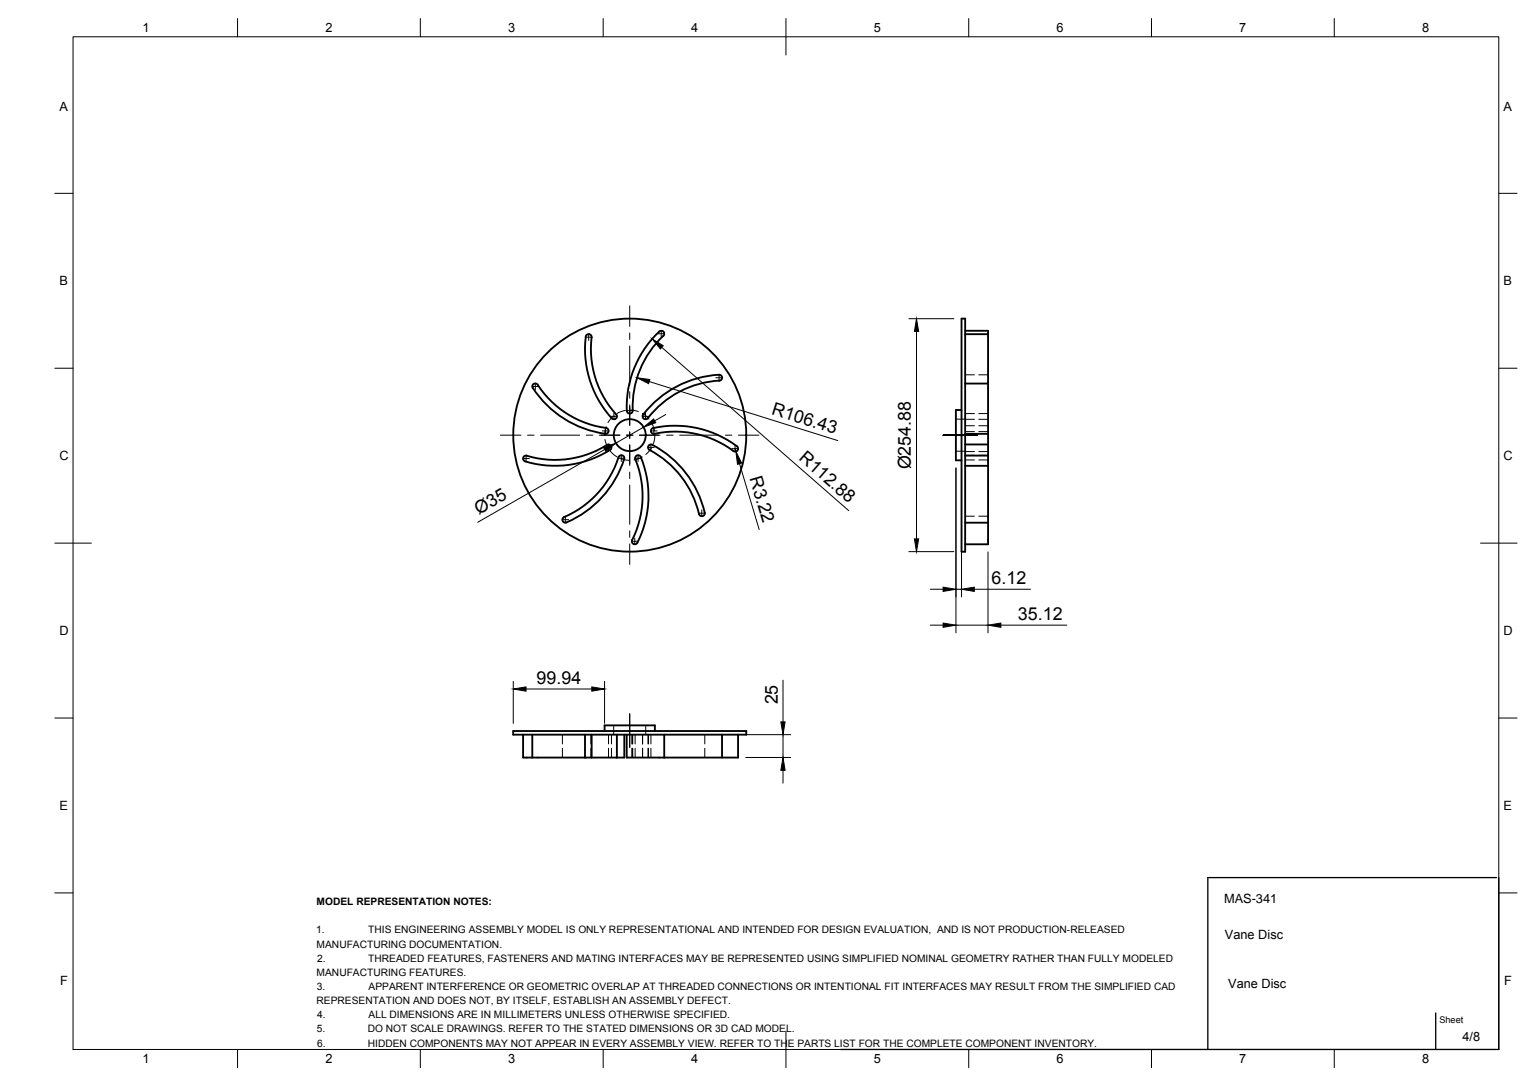
ISO-10303-21;
HEADER;
FILE_DESCRIPTION (('STEP AP214'),
    '1' );
FILE_NAME ('Vane Disc.step',
    '2026-10-08T00:39:10',
    ( '' ),
    ( '' ),
    'SwSTEP 2.0',
    'SolidWorks 2025',
    '' );
FILE_SCHEMA (( 'AUTOMOTIVE_DESIGN' ));
ENDSEC;

DATA;
#15=VECTOR ( 'NONE', #9741, 1000.000000000000000 ) ;
#47=AXIS2_PLACEMENT_3D ( 'NONE', #14477, #18892, #8730 ) ;
#49=ORIENTED_EDGE ( 'NONE', *, *, #19031, .T. ) ;
#59=LINE ( 'NONE', #18583, #13084 ) ;
#66=ORIENTED_EDGE ( 'NONE', *, *, #9551, .T. ) ;
#69=CARTESIAN_POINT ( 'NONE',  ( 57.41881860123199743, 83.27814316901175573, 14.88498244535504966 ) ) ;
#78=DIRECTION ( 'NONE',  ( 0.4999999999999920619, -0.8660254037844431485, -3.488064225688951427E-15 ) ) ;
#89=CARTESIAN_POINT ( 'NONE',  ( 9.176097008933345123, -25.21111933077053990, 14.88498244535538895 ) ) ;
#105=ADVANCED_FACE ( 'NONE', ( #15832 ), #1708, .T. ) ;
#111=FACE_OUTER_BOUND ( 'NONE', #19672, .T. ) ;
#131=DIRECTION ( 'NONE',  ( -0.1736481776669408228, -0.9848077530122062440, 2.152196535136390085E-15 ) ) ;
#138=CARTESIAN_POINT ( 'NONE',  ( -19.79297637435821500, 18.57624240429758800, 39.88498244535558968 ) ) ;
#141=VERTEX_POINT ( 'NONE', #14296 ) ;
#193=ORIENTED_EDGE ( 'NONE', *, *, #1304, .F. ) ;
#227=CIRCLE ( 'NONE', #11655, 3.224098631618461663 ) ;
#235=DIRECTION ( 'NONE',  ( 6.982962677686266711E-15, -0.000000000000000000, 1.000000000000000000 ) ) ;
#236=VECTOR ( 'NONE', #1051, 1000.000000000000000 ) ;
#239=CARTESIAN_POINT ( 'NONE',  ( 23.23469325536214214, -13.41455640552199924, 14.88498244535528947 ) ) ;
#259=PLANE ( 'NONE',  #6247 ) ;
#283=DIRECTION ( 'NONE',  ( 6.982962677686266711E-15, -0.000000000000000000, 1.000000000000000000 ) ) ;
#295=VERTEX_POINT ( 'NONE', #16702 ) ;
#302=CIRCLE ( 'NONE', #17951, 3.224098631618462552 ) ;
#306=LINE ( 'NONE', #12370, #13574 ) ;
#313=FACE_OUTER_BOUND ( 'NONE', #5653, .T. ) ;
#315=VERTEX_POINT ( 'NONE', #3550 ) ;
#316=DIRECTION ( 'NONE',  ( -1.000000000000000000, 0.000000000000000000, 6.976128451377902853E-15 ) ) ;
#334=CARTESIAN_POINT ( 'NONE',  ( 113.3640620605769413, -25.59923667990641150, 14.88498244535466064 ) ) ;
#354=CIRCLE ( 'NONE', #18993, 3.224098631618460331 ) ;
#362=DIRECTION ( 'NONE',  ( 6.982962677686266711E-15, -0.000000000000000000, 1.000000000000000000 ) ) ;
#368=ORIENTED_EDGE ( 'NONE', *, *, #19103, .F. ) ;
#379=DIRECTION ( 'NONE',  ( -6.982962677686266711E-15, 0.000000000000000000, -1.000000000000000000 ) ) ;
#390=CYLINDRICAL_SURFACE ( 'NONE', #8511, 3.224098631618460331 ) ;
#428=AXIS2_PLACEMENT_3D ( 'NONE', #8906, #8812, #13303 ) ;
#429=AXIS2_PLACEMENT_3D ( 'NONE', #16436, #7119, #13337 ) ;
#441=FACE_OUTER_BOUND ( 'NONE', #8088, .T. ) ;
#446=CARTESIAN_POINT ( 'NONE',  ( 19.63382932406841519, 18.38657833536341357, 39.88498244535531967 ) ) ;
#451=AXIS2_PLACEMENT_3D ( 'NONE', #4114, #2798, #845 ) ;
#456=DIRECTION ( 'NONE',  ( -0.7660444431189771253, 0.6427876096865404731, 5.349259755748777816E-15 ) ) ;
#460=AXIS2_PLACEMENT_3D ( 'NONE', #12907, #17728, #3504 ) ;
#465=CIRCLE ( 'NONE', #17772, 3.224098631618455890 ) ;
#466=FACE_OUTER_BOUND ( 'NONE', #14778, .T. ) ;
#478=EDGE_CURVE ( 'NONE', #6273, #3496, #1532, .T. ) ;
#485=CYLINDRICAL_SURFACE ( 'NONE', #1937, 3.224098631618460331 ) ;
#501=CIRCLE ( 'NONE', #1476, 17.50000000000000355 ) ;
#504=AXIS2_PLACEMENT_3D ( 'NONE', #6795, #13106, #738 ) ;
#520=EDGE_CURVE ( 'NONE', #7250, #912, #6769, .T. ) ;
#528=EDGE_LOOP ( 'NONE', ( #18695, #4336, #8989, #6164 ) ) ;
#533=AXIS2_PLACEMENT_3D ( 'NONE', #16138, #2125, #78 ) ;
#538=DIRECTION ( 'NONE',  ( 1.000000000000000000, 0.000000000000000000, -6.994638739193269649E-15 ) ) ;
#562=CARTESIAN_POINT ( 'NONE',  ( -32.30548103355237544, 113.3261241031799926, 14.88498244535567672 ) ) ;
#568=LINE ( 'NONE', #2209, #10145 ) ;
#582=AXIS2_PLACEMENT_3D ( 'NONE', #17065, #9285, #15422 ) ;
#612=LINE ( 'NONE', #19529, #7209 ) ;
#613=DIRECTION ( 'NONE',  ( -6.982962677686266711E-15, 0.000000000000000000, -1.000000000000000000 ) ) ;
#619=ORIENTED_EDGE ( 'NONE', *, *, #10225, .F. ) ;
#640=LINE ( 'NONE', #13102, #7507 ) ;
#641=CARTESIAN_POINT ( 'NONE',  ( -113.3514208120937781, -17.29894464209964866, 14.88498244535624337 ) ) ;
#643=( NAMED_UNIT ( * ) SI_UNIT ( $, .STERADIAN. ) SOLID_ANGLE_UNIT ( ) );
#650=DIRECTION ( 'NONE',  ( -6.982962677686266711E-15, 0.000000000000000000, -1.000000000000000000 ) ) ;
#691=CARTESIAN_POINT ( 'NONE',  ( -34.51244174799990816, 110.9757759606085017, 14.88498244535569093 ) ) ;
#692=DIRECTION ( 'NONE',  ( -0.7660444431189766812, 0.6427876096865408062, 4.304393070272782536E-15 ) ) ;
#724=CIRCLE ( 'NONE', #19044, 3.224098631618458999 ) ;
#732=AXIS2_PLACEMENT_3D ( 'NONE', #11861, #13300, #19653 ) ;
#734=DIRECTION ( 'NONE',  ( -6.982962677686265922E-15, -1.972152263052529514E-31, -1.000000000000000000 ) ) ;
#735=CARTESIAN_POINT ( 'NONE',  ( 23.23469325536214214, -13.41455640552199924, 14.88498244535528947 ) ) ;
#738=DIRECTION ( 'NONE',  ( 0.5000000000000038858, 0.8660254037844363761, -3.520662956770155909E-15 ) ) ;
#745=EDGE_CURVE ( 'NONE', #1745, #14667, #18421, .T. ) ;
#747=ORIENTED_EDGE ( 'NONE', *, *, #8839, .T. ) ;
#749=CARTESIAN_POINT ( 'NONE',  ( 92.34802049131684498, -66.64338626758360817, 14.88498244535480630 ) ) ;
#754=DIRECTION ( 'NONE',  ( 6.982962677686266711E-15, -0.000000000000000000, 1.000000000000000000 ) ) ;
#759=CARTESIAN_POINT ( 'NONE',  ( -26.42151830275515323, 4.658826548058537576, 14.88498244535563586 ) ) ;
#790=CARTESIAN_POINT ( 'NONE',  ( -63.98537287693023501, 94.20918150411493741, 39.88498244535590231 ) ) ;
#792=ORIENTED_EDGE ( 'NONE', *, *, #6721, .T. ) ;
#797=CARTESIAN_POINT ( 'NONE',  ( -9.176097008933940202, -25.21111933077039069, 39.88498244535551862 ) ) ;
#807=VERTEX_POINT ( 'NONE', #18628 ) ;
#818=VERTEX_POINT ( 'NONE', #9309 ) ;
#831=FACE_OUTER_BOUND ( 'NONE', #15190, .T. ) ;
#845=DIRECTION ( 'NONE',  ( 1.000000000000000000, 0.000000000000000000, -6.994638739193269649E-15 ) ) ;
#850=CARTESIAN_POINT ( 'NONE',  ( -63.98537287693023501, 94.20918150411493741, 39.88498244535590231 ) ) ;
#851=ADVANCED_FACE ( 'NONE', ( #5221 ), #6350, .T. ) ;
#863=ORIENTED_EDGE ( 'NONE', *, *, #8888, .F. ) ;
#891=CIRCLE ( 'NONE', #13620, 3.224098631618461663 ) ;
#895=AXIS2_PLACEMENT_3D ( 'NONE', #13323, #2501, #8636 ) ;
#896=EDGE_CURVE ( 'NONE', #12923, #1501, #465, .T. ) ;
#904=EDGE_CURVE ( 'NONE', #2440, #7038, #2047, .T. ) ;
#908=DIRECTION ( 'NONE',  ( 6.982962677686266711E-15, -0.000000000000000000, 1.000000000000000000 ) ) ;
#912=VERTEX_POINT ( 'NONE', #10300 ) ;
#931=CARTESIAN_POINT ( 'NONE',  ( -20.01059462374426445, -13.41455640552162443, 14.88498244535559323 ) ) ;
#936=DIRECTION ( 'NONE',  ( -0.7660444431189770143, 0.6427876096865405842, 5.348151281215662765E-15 ) ) ;
#965=ORIENTED_EDGE ( 'NONE', *, *, #16251, .F. ) ;
#979=AXIS2_PLACEMENT_3D ( 'NONE', #2375, #18027, #5444 ) ;
#981=CARTESIAN_POINT ( 'NONE',  ( 112.4320812185962524, -22.51277856475483574, 14.88498244535466775 ) ) ;
#994=LINE ( 'NONE', #7047, #13321 ) ;
#996=FACE_OUTER_BOUND ( 'NONE', #16761, .T. ) ;
#1003=CARTESIAN_POINT ( 'NONE',  ( -49.59485801383857506, -102.5175491340983882, 14.88498244535579929 ) ) ;
#1008=DIRECTION ( 'NONE',  ( -6.982962677686268288E-15, 3.944304526105059903E-31, -1.000000000000000000 ) ) ;
#1009=ORIENTED_EDGE ( 'NONE', *, *, #7477, .F. ) ;
#1017=VECTOR ( 'NONE', #3317, 1000.000000000000000 ) ;
#1024=CARTESIAN_POINT ( 'NONE',  ( 25.98398601615827985, 7.853099154550822192, 14.88498244535527171 ) ) ;
#1045=ORIENTED_EDGE ( 'NONE', *, *, #5358, .T. ) ;
#1051=DIRECTION ( 'NONE',  ( 6.982962677686266711E-15, -0.000000000000000000, 1.000000000000000000 ) ) ;
#1056=CIRCLE ( 'NONE', #8250, 3.224098631618458555 ) ;
#1060=CIRCLE ( 'NONE', #5338, 27.50000000000000355 ) ;
#1065=AXIS2_PLACEMENT_3D ( 'NONE', #69, #12331, #10906 ) ;
#1066=DIRECTION ( 'NONE',  ( -1.000000000000000000, 0.000000000000000000, 0.000000000000000000 ) ) ;
#1067=CARTESIAN_POINT ( 'NONE',  ( -49.59485801383857506, -102.5175491340983882, 14.88498244535579929 ) ) ;
#1079=CIRCLE ( 'NONE', #19402, 3.224098631618458999 ) ;
#1080=VERTEX_POINT ( 'NONE', #12131 ) ;
#1084=MANIFOLD_SOLID_BREP ( 'Boss-Extrude13', #11640 ) ;
#1110=ORIENTED_EDGE ( 'NONE', *, *, #2464, .F. ) ;
#1134=CARTESIAN_POINT ( 'NONE',  ( -2.647132857508548209, -114.6332882433608376, 14.88498244535546888 ) ) ;
#1136=ORIENTED_EDGE ( 'NONE', *, *, #18917, .F. ) ;
#1170=DIRECTION ( 'NONE',  ( 1.000000000000000000, 0.000000000000000000, -6.977185866873308817E-15 ) ) ;
#1189=AXIS2_PLACEMENT_3D ( 'NONE', #2625, #2520, #15088 ) ;
#1198=CIRCLE ( 'NONE', #19820, 3.224098631618463440 ) ;
#1200=DIRECTION ( 'NONE',  ( 1.000000000000000000, 0.000000000000000000, -6.994638739193269649E-15 ) ) ;
#1209=CARTESIAN_POINT ( 'NONE',  ( -1.396592535537253342E-14, 0.000000000000000000, 39.88498244535545467 ) ) ;
#1225=DIRECTION ( 'NONE',  ( 0.9396926207859057634, -0.3420201433256758183, -6.456589605409169860E-15 ) ) ;
#1235=ORIENTED_EDGE ( 'NONE', *, *, #20238, .T. ) ;
#1236=CYLINDRICAL_SURFACE ( 'NONE', #15630, 112.8770930172170210 ) ;
#1244=AXIS2_PLACEMENT_3D ( 'NONE', #14765, #2203, #19186 ) ;
#1254=DIRECTION ( 'NONE',  ( 6.982962677686266711E-15, 0.000000000000000000, 1.000000000000000000 ) ) ;
#1261=CIRCLE ( 'NONE', #14662, 106.4288957539801004 ) ;
#1264=AXIS2_PLACEMENT_3D ( 'NONE', #6211, #1494, #1695 ) ;
#1290=CARTESIAN_POINT ( 'NONE',  ( 27.50000000000001776, 3.367778697655222096E-15, 49.99999999999998579 ) ) ;
#1301=DIRECTION ( 'NONE',  ( 6.982962677686266711E-15, -0.000000000000000000, 1.000000000000000000 ) ) ;
#1304=EDGE_CURVE ( 'NONE', #6273, #295, #16535, .T. ) ;
#1308=ORIENTED_EDGE ( 'NONE', *, *, #4869, .T. ) ;
#1311=LINE ( 'NONE', #8969, #8332 ) ;
#1316=CARTESIAN_POINT ( 'NONE',  ( -27.49999999999998934, 0.000000000000000000, 49.99999999999998579 ) ) ;
#1331=ORIENTED_EDGE ( 'NONE', *, *, #4320, .F. ) ;
#1340=CYLINDRICAL_SURFACE ( 'NONE', #18052, 3.224098631618460331 ) ;
#1361=CYLINDRICAL_SURFACE ( 'NONE', #13666, 3.224098631618460331 ) ;
#1371=EDGE_CURVE ( 'NONE', #7864, #8547, #19790, .T. ) ;
#1384=CARTESIAN_POINT ( 'NONE',  ( 113.5802308907675666, 8.308367629983374414, 14.88498244535465709 ) ) ;
#1401=VERTEX_POINT ( 'NONE', #10676 ) ;
#1411=ORIENTED_EDGE ( 'NONE', *, *, #10835, .F. ) ;
#1427=EDGE_LOOP ( 'NONE', ( #19804, #8340, #5647, #20218 ) ) ;
#1433=ORIENTED_EDGE ( 'NONE', *, *, #6415, .F. ) ;
#1461=CARTESIAN_POINT ( 'NONE',  ( -14.69786621328394283, 22.52834316112731017, 39.88498244535555415 ) ) ;
#1476=AXIS2_PLACEMENT_3D ( 'NONE', #15111, #17998, #7440 ) ;
#1494=DIRECTION ( 'NONE',  ( 6.982962677686266711E-15, -0.000000000000000000, 1.000000000000000000 ) ) ;
#1495=LINE ( 'NONE', #17151, #9162 ) ;
#1501=VERTEX_POINT ( 'NONE', #15497 ) ;
#1506=ORIENTED_EDGE ( 'NONE', *, *, #8714, .T. ) ;
#1515=AXIS2_PLACEMENT_3D ( 'NONE', #7804, #13076, #3208 ) ;
#1532=CIRCLE ( 'NONE', #13602, 127.4413876050234649 ) ;
#1543=EDGE_CURVE ( 'NONE', #6114, #17930, #5067, .T. ) ;
#1553=CARTESIAN_POINT ( 'NONE',  ( -81.99056186900673993, -84.64042930812179577, 14.88498244535602488 ) ) ;
#1600=ORIENTED_EDGE ( 'NONE', *, *, #3125, .F. ) ;
#1630=CARTESIAN_POINT ( 'NONE',  ( -75.71267875615025389, -86.11264925328200093, 14.88498244535597870 ) ) ;
#1633=DIRECTION ( 'NONE',  ( 6.982962677686266711E-15, -0.000000000000000000, 1.000000000000000000 ) ) ;
#1647=LINE ( 'NONE', #6357, #17013 ) ;
#1648=DIRECTION ( 'NONE',  ( -6.982962677686266711E-15, 0.000000000000000000, -1.000000000000000000 ) ) ;
#1654=DIRECTION ( 'NONE',  ( 6.982962677686266711E-15, -0.000000000000000000, 1.000000000000000000 ) ) ;
#1671=CARTESIAN_POINT ( 'NONE',  ( -2.300765332208190905, -116.0870680293436408, 39.88498244535547599 ) ) ;
#1676=CARTESIAN_POINT ( 'NONE',  ( 27.50000000000001776, 3.367778697655222096E-15, 43.88498244535526993 ) ) ;
#1694=DIRECTION ( 'NONE',  ( 6.982962677686266711E-15, -0.000000000000000000, 1.000000000000000000 ) ) ;
#1695=DIRECTION ( 'NONE',  ( 1.000000000000000000, 0.000000000000000000, -6.977185866873308817E-15 ) ) ;
#1696=CARTESIAN_POINT ( 'NONE',  ( -19.79297637435836421, 18.57624240429761642, 14.88498244535559145 ) ) ;
#1698=ORIENTED_EDGE ( 'NONE', *, *, #16107, .F. ) ;
#1708=CYLINDRICAL_SURFACE ( 'NONE', #3475, 3.224098631618460331 ) ;
#1727=AXIS2_PLACEMENT_3D ( 'NONE', #16670, #1633, #18506 ) ;
#1733=DIRECTION ( 'NONE',  ( 1.000000000000000000, 0.000000000000000000, -6.977185866873309606E-15 ) ) ;
#1743=DIRECTION ( 'NONE',  ( 6.982962677686266711E-15, -0.000000000000000000, 1.000000000000000000 ) ) ;
#1745=VERTEX_POINT ( 'NONE', #562 ) ;
#1748=CARTESIAN_POINT ( 'NONE',  ( -6.191009641800430785, -26.42934155884822900, 14.88498244535549375 ) ) ;
#1760=ORIENTED_EDGE ( 'NONE', *, *, #17363, .F. ) ;
#1763=MECHANICAL_DESIGN_GEOMETRIC_PRESENTATION_REPRESENTATION('',(#18100),#5359);
#1777=CIRCLE ( 'NONE', #8629, 3.224098631618458999 ) ;
#1797=DIRECTION ( 'NONE',  ( 0.5000000000000038858, 0.8660254037844362651, -3.503961184244744203E-15 ) ) ;
#1799=FACE_BOUND ( 'NONE', #7536, .T. ) ;
#1801=DIRECTION ( 'NONE',  ( 6.982962677686266711E-15, -0.000000000000000000, 1.000000000000000000 ) ) ;
#1807=VERTEX_POINT ( 'NONE', #16606 ) ;
#1814=AXIS2_PLACEMENT_3D ( 'NONE', #14717, #19236, #2052 ) ;
#1824=AXIS2_PLACEMENT_3D ( 'NONE', #9990, #3945, #13342 ) ;
#1830=ORIENTED_EDGE ( 'NONE', *, *, #7477, .T. ) ;
#1839=ORIENTED_EDGE ( 'NONE', *, *, #16386, .F. ) ;
#1862=VERTEX_POINT ( 'NONE', #4019 ) ;
#1874=VECTOR ( 'NONE', #18951, 1000.000000000000000 ) ;
#1877=FACE_OUTER_BOUND ( 'NONE', #6342, .T. ) ;
#1891=EDGE_CURVE ( 'NONE', #1401, #4820, #9815, .T. ) ;
#1898=CARTESIAN_POINT ( 'NONE',  ( -81.99056186900673993, -84.64042930812179577, 14.88498244535602488 ) ) ;
#1900=DIRECTION ( 'NONE',  ( -0.1736481776669404620, -0.9848077530122062440, 1.229460064647279239E-15 ) ) ;
#1902=CIRCLE ( 'NONE', #9740, 3.224098631618460331 ) ;
#1911=EDGE_LOOP ( 'NONE', ( #19538, #3190 ) ) ;
#1918=CIRCLE ( 'NONE', #18576, 3.224098631618463440 ) ;
#1937=AXIS2_PLACEMENT_3D ( 'NONE', #10093, #14596, #6729 ) ;
#1944=LINE ( 'NONE', #8173, #2255 ) ;
#1946=CARTESIAN_POINT ( 'NONE',  ( 1.396592535537252080E-14, 0.000000000000000000, 49.99999999999998579 ) ) ;
#1956=DIRECTION ( 'NONE',  ( -6.982962677686266711E-15, 0.000000000000000000, -1.000000000000000000 ) ) ;
#1980=AXIS2_PLACEMENT_3D ( 'NONE', #4506, #9206, #7367 ) ;
#1986=PLANE ( 'NONE',  #4620 ) ;
#1994=VERTEX_POINT ( 'NONE', #11245 ) ;
#2003=CIRCLE ( 'NONE', #17696, 3.224098631618460331 ) ;
#2009=ORIENTED_EDGE ( 'NONE', *, *, #9610, .T. ) ;
#2014=VERTEX_POINT ( 'NONE', #641 ) ;
#2023=DIRECTION ( 'NONE',  ( 1.000000000000000000, 0.000000000000000000, -6.977185866873308817E-15 ) ) ;
#2024=ORIENTED_EDGE ( 'NONE', *, *, #9144, .F. ) ;
#2027=CARTESIAN_POINT ( 'NONE',  ( 103.2967819461769921, 53.25886146954521649, 39.88498244535472992 ) ) ;
#2034=DIRECTION ( 'NONE',  ( 6.982962677686266711E-15, -0.000000000000000000, 1.000000000000000000 ) ) ;
#2036=DIRECTION ( 'NONE',  ( -6.982962677686266711E-15, 0.000000000000000000, -1.000000000000000000 ) ) ;
#2047=LINE ( 'NONE', #8277, #14496 ) ;
#2050=EDGE_CURVE ( 'NONE', #16647, #4108, #4200, .T. ) ;
#2052=DIRECTION ( 'NONE',  ( -1.000000000000000000, 0.000000000000000000, 6.969309079188926949E-15 ) ) ;
#2053=CARTESIAN_POINT ( 'NONE',  ( -12.16118437606778535, -23.99289710269258080, 14.88498244535553461 ) ) ;
#2069=ORIENTED_EDGE ( 'NONE', *, *, #9873, .T. ) ;
#2086=AXIS2_PLACEMENT_3D ( 'NONE', #790, #13357, #2531 ) ;
#2089=DIRECTION ( 'NONE',  ( -6.982962677686266711E-15, 0.000000000000000000, -1.000000000000000000 ) ) ;
#2115=CIRCLE ( 'NONE', #14846, 112.8770930172170353 ) ;
#2125=DIRECTION ( 'NONE',  ( 6.982962677686266711E-15, 0.000000000000000000, 1.000000000000000000 ) ) ;
#2138=EDGE_LOOP ( 'NONE', ( #12512, #19684, #12449, #17623, #12034 ) ) ;
#2156=CYLINDRICAL_SURFACE ( 'NONE', #1515, 112.8770930172170068 ) ;
#2159=DIRECTION ( 'NONE',  ( 1.000000000000000000, 0.000000000000000000, -6.977185866873308817E-15 ) ) ;
#2163=DIRECTION ( 'NONE',  ( 1.000000000000000000, 0.000000000000000000, -6.994638739193269649E-15 ) ) ;
#2170=VERTEX_POINT ( 'NONE', #15944 ) ;
#2171=AXIS2_PLACEMENT_3D ( 'NONE', #7203, #10261, #7102 ) ;
#2184=VERTEX_POINT ( 'NONE', #17783 ) ;
#2195=CIRCLE ( 'NONE', #1189, 3.224098631618460331 ) ;
#2199=DIRECTION ( 'NONE',  ( 6.982962677686266711E-15, -0.000000000000000000, 1.000000000000000000 ) ) ;
#2203=DIRECTION ( 'NONE',  ( 6.982962677686266711E-15, -0.000000000000000000, 1.000000000000000000 ) ) ;
#2209=CARTESIAN_POINT ( 'NONE',  ( 6.106329265062790945, -26.19668413589285194, 14.88498244535541026 ) ) ;
#2212=VECTOR ( 'NONE', #12651, 1000.000000000000000 ) ;
#2213=ORIENTED_EDGE ( 'NONE', *, *, #9199, .F. ) ;
#2214=AXIS2_PLACEMENT_3D ( 'NONE', #13685, #4382, #20133 ) ;
#2217=ORIENTED_EDGE ( 'NONE', *, *, #7018, .F. ) ;
#2220=EDGE_LOOP ( 'NONE', ( #965, #6524, #11975, #17424 ) ) ;
#2227=ORIENTED_EDGE ( 'NONE', *, *, #10835, .T. ) ;
#2251=EDGE_CURVE ( 'NONE', #12128, #7331, #354, .T. ) ;
#2255=VECTOR ( 'NONE', #17295, 1000.000000000000000 ) ;
#2256=AXIS2_PLACEMENT_3D ( 'NONE', #2903, #17019, #2801 ) ;
#2259=DIRECTION ( 'NONE',  ( 1.000000000000000000, 0.000000000000000000, -6.976128451377902853E-15 ) ) ;
#2261=ORIENTED_EDGE ( 'NONE', *, *, #19165, .T. ) ;
#2262=CARTESIAN_POINT ( 'NONE',  ( 43.41157826374501383, -91.36522714846361737, 14.88498244535515092 ) ) ;
#2286=DIRECTION ( 'NONE',  ( -0.1736481776669280275, 0.9848077530122084644, 1.076098267568195831E-15 ) ) ;
#2287=FACE_OUTER_BOUND ( 'NONE', #13566, .T. ) ;
#2292=EDGE_LOOP ( 'NONE', ( #11795, #6552, #5825, #9650, #2390 ) ) ;
#2308=DIRECTION ( 'NONE',  ( -6.982962677686266711E-15, 0.000000000000000000, -1.000000000000000000 ) ) ;
#2334=LINE ( 'NONE', #5907, #5129 ) ;
#2341=VERTEX_POINT ( 'NONE', #5591 ) ;
#2356=PLANE ( 'NONE',  #15439 ) ;
#2368=ORIENTED_EDGE ( 'NONE', *, *, #3905, .T. ) ;
#2372=AXIS2_PLACEMENT_3D ( 'NONE', #11461, #15974, #14437 ) ;
#2375=CARTESIAN_POINT ( 'NONE',  ( 26.42151830275502178, 4.658826548058130790, 39.88498244535526993 ) ) ;
#2378=( NAMED_UNIT ( * ) PLANE_ANGLE_UNIT ( ) SI_UNIT ( $, .RADIAN. ) );
#2385=VECTOR ( 'NONE', #9210, 1000.000000000000000 ) ;
#2390=ORIENTED_EDGE ( 'NONE', *, *, #8482, .T. ) ;
#2409=VERTEX_POINT ( 'NONE', #12117 ) ;
#2426=VERTEX_POINT ( 'NONE', #17253 ) ;
#2432=CARTESIAN_POINT ( 'NONE',  ( -78.85162031257850401, -85.37653928070189124, 14.88498244535600357 ) ) ;
#2440=VERTEX_POINT ( 'NONE', #1290 ) ;
#2452=FACE_OUTER_BOUND ( 'NONE', #7683, .T. ) ;
#2464=EDGE_CURVE ( 'NONE', #1862, #16627, #2003, .T. ) ;
#2466=CARTESIAN_POINT ( 'NONE',  ( -23.23469325536272478, -13.41455640552162443, 14.88498244535561454 ) ) ;
#2476=DIRECTION ( 'NONE',  ( 0.5000000000000044409, 0.8660254037844360431, -3.228294802704586902E-15 ) ) ;
#2477=CARTESIAN_POINT ( 'NONE',  ( -19.79297637435836421, 18.57624240429761642, 14.88498244535559145 ) ) ;
#2482=DIRECTION ( 'NONE',  ( -6.982962677686266711E-15, 0.000000000000000000, -1.000000000000000000 ) ) ;
#2493=LINE ( 'NONE', #14864, #17654 ) ;
#2499=EDGE_CURVE ( 'NONE', #6452, #10937, #9506, .T. ) ;
#2501=DIRECTION ( 'NONE',  ( 6.982962677686266711E-15, 0.000000000000000000, 1.000000000000000000 ) ) ;
#2504=VECTOR ( 'NONE', #6931, 1000.000000000000000 ) ;
#2506=AXIS2_PLACEMENT_3D ( 'NONE', #2466, #14836, #18114 ) ;
#2513=DIRECTION ( 'NONE',  ( 6.982962677686266711E-15, -0.000000000000000000, 1.000000000000000000 ) ) ;
#2520=DIRECTION ( 'NONE',  ( -6.982962677686266711E-15, 0.000000000000000000, -1.000000000000000000 ) ) ;
#2531=DIRECTION ( 'NONE',  ( -0.7660444431189770143, 0.6427876096865404731, 5.348151281215661977E-15 ) ) ;
#2532=EDGE_LOOP ( 'NONE', ( #16841, #13833, #9327, #7473 ) ) ;
#2538=CIRCLE ( 'NONE', #8424, 3.224098631618455890 ) ;
#2555=VERTEX_POINT ( 'NONE', #14581 ) ;
#2556=CIRCLE ( 'NONE', #18580, 106.4288957539801004 ) ;
#2562=CARTESIAN_POINT ( 'NONE',  ( 3.304959094393253416, 31.03941509555038181, 14.88498244535543158 ) ) ;
#2580=DIRECTION ( 'NONE',  ( -1.000000000000000000, 0.000000000000000000, 6.994638739193269649E-15 ) ) ;
#2589=EDGE_CURVE ( 'NONE', #19558, #4614, #11097, .T. ) ;
#2593=CARTESIAN_POINT ( 'NONE',  ( -109.5721339228237667, 31.03941509555038181, 14.88498244535621851 ) ) ;
#2597=DIRECTION ( 'NONE',  ( 6.982962677686266711E-15, 0.000000000000000000, 1.000000000000000000 ) ) ;
#2614=EDGE_LOOP ( 'NONE', ( #3626, #14039, #11730, #7222 ) ) ;
#2623=LINE ( 'NONE', #6930, #20205 ) ;
#2625=CARTESIAN_POINT ( 'NONE',  ( -17.24542129382105315, 20.55229278271246329, 39.88498244535557546 ) ) ;
#2628=CIRCLE ( 'NONE', #6555, 112.8770930172170495 ) ;
#2632=DIRECTION ( 'NONE',  ( 0.000000000000000000, 0.000000000000000000, 1.000000000000000000 ) ) ;
#2634=LINE ( 'NONE', #8859, #18820 ) ;
#2636=EDGE_LOOP ( 'NONE', ( #12071, #6685, #2683, #19660 ) ) ;
#2652=DIRECTION ( 'NONE',  ( 6.982962677686266711E-15, -0.000000000000000000, 1.000000000000000000 ) ) ;
#2665=EDGE_CURVE ( 'NONE', #807, #11267, #3835, .T. ) ;
#2670=ORIENTED_EDGE ( 'NONE', *, *, #11507, .T. ) ;
#2676=CARTESIAN_POINT ( 'NONE',  ( -14.02132266220259460, 20.55229278271246329, 39.88498244535555415 ) ) ;
#2679=DIRECTION ( 'NONE',  ( -0.7660444431189766812, 0.6427876096865408062, 5.380491337840978959E-15 ) ) ;
#2682=LINE ( 'NONE', #19756, #12827 ) ;
#2683=ORIENTED_EDGE ( 'NONE', *, *, #11372, .F. ) ;
#2700=VECTOR ( 'NONE', #10838, 1000.000000000000000 ) ;
#2707=ORIENTED_EDGE ( 'NONE', *, *, #11874, .T. ) ;
#2722=DIRECTION ( 'NONE',  ( -6.982962677686266711E-15, 0.000000000000000000, -1.000000000000000000 ) ) ;
#2727=EDGE_CURVE ( 'NONE', #10937, #7509, #17898, .T. ) ;
#2738=FACE_OUTER_BOUND ( 'NONE', #2292, .T. ) ;
#2782=EDGE_CURVE ( 'NONE', #818, #10937, #15071, .T. ) ;
#2786=VERTEX_POINT ( 'NONE', #5774 ) ;
#2798=DIRECTION ( 'NONE',  ( 6.982962677686266711E-15, -0.000000000000000000, 1.000000000000000000 ) ) ;
#2801=DIRECTION ( 'NONE',  ( -0.7660444431189858960, -0.6427876096865299260, 5.348151281215661977E-15 ) ) ;
#2817=ORIENTED_EDGE ( 'NONE', *, *, #18917, .T. ) ;
#2823=DIRECTION ( 'NONE',  ( 0.9396926207859058744, -0.3420201433256757628, -6.568644312862837946E-15 ) ) ;
#2832=DIRECTION ( 'NONE',  ( 0.9396926207859057634, -0.3420201433256758183, -6.456589605409169860E-15 ) ) ;
#2834=ADVANCED_FACE ( 'NONE', ( #15591 ), #4751, .T. ) ;
#2860=FACE_BOUND ( 'NONE', #7834, .T. ) ;
#2880=DIRECTION ( 'NONE',  ( 6.982962677686266711E-15, -0.000000000000000000, 1.000000000000000000 ) ) ;
#2903=CARTESIAN_POINT ( 'NONE',  ( -103.8888757476053541, -46.65403860089418941, 14.88498244535617765 ) ) ;
#2917=AXIS2_PLACEMENT_3D ( 'NONE', #13299, #10333, #11860 ) ;
#2918=VERTEX_POINT ( 'NONE', #17128 ) ;
#2929=CARTESIAN_POINT ( 'NONE',  ( 9.176097008933345123, -25.21111933077053990, 14.88498244535538895 ) ) ;
#2930=FACE_OUTER_BOUND ( 'NONE', #5894, .T. ) ;
#2935=DIRECTION ( 'NONE',  ( 6.982962677686266711E-15, -0.000000000000000000, 1.000000000000000000 ) ) ;
#2940=DIRECTION ( 'NONE',  ( 0.9396926207859104263, 0.3420201433256629953, -6.562243095054850434E-15 ) ) ;
#2948=FILL_AREA_STYLE_COLOUR ( '', #12204 ) ;
#2982=CARTESIAN_POINT ( 'NONE',  ( -113.3514208120937781, -17.29894464209964866, 14.88498244535624337 ) ) ;
#2987=ADVANCED_FACE ( 'NONE', ( #11483, #9746 ), #1986, .T. ) ;
#3002=EDGE_CURVE ( 'NONE', #3496, #6917, #17341, .T. ) ;
#3036=CARTESIAN_POINT ( 'NONE',  ( 9.176097008933519206, -25.21111933077053990, 39.88498244535539072 ) ) ;
#3046=ADVANCED_FACE ( 'NONE', ( #1877 ), #3212, .T. ) ;
#3054=DIRECTION ( 'NONE',  ( -0.1736481776669405452, -0.9848077530122062440, 1.214091813839188261E-15 ) ) ;
#3056=CYLINDRICAL_SURFACE ( 'NONE', #11893, 3.224098631618457667 ) ;
#3068=CARTESIAN_POINT ( 'NONE',  ( 113.3640620605769413, -25.59923667990641150, 14.88498244535466064 ) ) ;
#3077=CIRCLE ( 'NONE', #8939, 3.224098631618458555 ) ;
#3088=VERTEX_POINT ( 'NONE', #4961 ) ;
#3099=ORIENTED_EDGE ( 'NONE', *, *, #14653, .F. ) ;
#3116=VERTEX_POINT ( 'NONE', #5257 ) ;
#3119=EDGE_CURVE ( 'NONE', #9562, #315, #302, .T. ) ;
#3125=EDGE_CURVE ( 'NONE', #11508, #15057, #9778, .T. ) ;
#3134=DIRECTION ( 'NONE',  ( 1.000000000000000000, 0.000000000000000000, -6.969309079188926949E-15 ) ) ;
#3153=CYLINDRICAL_SURFACE ( 'NONE', #7761, 112.8770930172170210 ) ;
#3165=CIRCLE ( 'NONE', #14589, 3.224098631618458555 ) ;
#3190=ORIENTED_EDGE ( 'NONE', *, *, #7762, .T. ) ;
#3191=AXIS2_PLACEMENT_3D ( 'NONE', #9188, #5107, #10924 ) ;
#3194=AXIS2_PLACEMENT_3D ( 'NONE', #15486, #17025, #18351 ) ;
#3196=EDGE_LOOP ( 'NONE', ( #17005, #17105, #18751, #747, #18294, #2069 ) ) ;
#3202=VERTEX_POINT ( 'NONE', #2477 ) ;
#3208=DIRECTION ( 'NONE',  ( 1.000000000000000000, 0.000000000000000000, -6.977185866873309606E-15 ) ) ;
#3212=CYLINDRICAL_SURFACE ( 'NONE', #5592, 3.224098631618457667 ) ;
#3224=DIRECTION ( 'NONE',  ( 1.000000000000000000, 0.000000000000000000, -6.976128451377903642E-15 ) ) ;
#3227=DIRECTION ( 'NONE',  ( 1.000000000000000000, 0.000000000000000000, -6.994638739193269649E-15 ) ) ;
#3230=DIRECTION ( 'NONE',  ( 6.982962677686266711E-15, 0.000000000000000000, 1.000000000000000000 ) ) ;
#3237=ADVANCED_FACE ( 'NONE', ( #831 ), #6984, .T. ) ;
#3272=EDGE_CURVE ( 'NONE', #8591, #18684, #15440, .T. ) ;
#3278=DIRECTION ( 'NONE',  ( 1.000000000000000000, 0.000000000000000000, -6.994638739193269649E-15 ) ) ;
#3284=DIRECTION ( 'NONE',  ( 6.982962677686266711E-15, -0.000000000000000000, 1.000000000000000000 ) ) ;
#3286=DIRECTION ( 'NONE',  ( -6.982962677686266711E-15, 0.000000000000000000, -1.000000000000000000 ) ) ;
#3291=CYLINDRICAL_SURFACE ( 'NONE', #13183, 106.4288957539801004 ) ;
#3312=DIRECTION ( 'NONE',  ( 1.000000000000000000, 0.000000000000000000, -6.976128451377902853E-15 ) ) ;
#3317=DIRECTION ( 'NONE',  ( 6.982962677686266711E-15, -0.000000000000000000, 1.000000000000000000 ) ) ;
#3319=ORIENTED_EDGE ( 'NONE', *, *, #2589, .F. ) ;
#3322=AXIS2_PLACEMENT_3D ( 'NONE', #13528, #18053, #16618 ) ;
#3337=PLANE ( 'NONE',  #9029 ) ;
#3339=ORIENTED_EDGE ( 'NONE', *, *, #9551, .F. ) ;
#3369=AXIS2_PLACEMENT_3D ( 'NONE', #8959, #1301, #5805 ) ;
#3375=CARTESIAN_POINT ( 'NONE',  ( -5.524863963826822655, -116.0870680293436408, 14.88498244535549020 ) ) ;
#3381=EDGE_CURVE ( 'NONE', #1807, #11267, #9004, .T. ) ;
#3383=AXIS2_PLACEMENT_3D ( 'NONE', #749, #2199, #19286 ) ;
#3423=ADVANCED_FACE ( 'NONE', ( #111 ), #3291, .F. ) ;
#3425=EDGE_LOOP ( 'NONE', ( #16382, #14638, #12899, #18330 ) ) ;
#3445=ORIENTED_EDGE ( 'NONE', *, *, #16774, .F. ) ;
#3459=CIRCLE ( 'NONE', #13569, 112.8770930172170210 ) ;
#3474=CARTESIAN_POINT ( 'NONE',  ( 25.98398601615845038, 7.853099154550832850, 39.88498244535526993 ) ) ;
#3475=AXIS2_PLACEMENT_3D ( 'NONE', #14393, #4992, #17061 ) ;
#3477=ORIENTED_EDGE ( 'NONE', *, *, #14791, .T. ) ;
#3480=AXIS2_PLACEMENT_3D ( 'NONE', #4157, #16644, #16452 ) ;
#3482=ADVANCED_FACE ( 'NONE', ( #313 ), #3592, .T. ) ;
#3488=CARTESIAN_POINT ( 'NONE',  ( -1.396592535537253342E-14, 0.000000000000000000, 39.88498244535545467 ) ) ;
#3496=VERTEX_POINT ( 'NONE', #11051 ) ;
#3504=DIRECTION ( 'NONE',  ( 0.4999999999999925060, -0.8660254037844429265, -4.304393070272789636E-15 ) ) ;
#3506=LINE ( 'NONE', #12910, #15 ) ;
#3547=ORIENTED_EDGE ( 'NONE', *, *, #1891, .T. ) ;
#3548=CIRCLE ( 'NONE', #14966, 3.224098631618461219 ) ;
#3550=CARTESIAN_POINT ( 'NONE',  ( 24.95276293194433492, -10.68636129284900704, 14.88498244535527881 ) ) ;
#3564=DIRECTION ( 'NONE',  ( 1.000000000000000000, 0.000000000000000000, -6.994638739193269649E-15 ) ) ;
#3592=CYLINDRICAL_SURFACE ( 'NONE', #9800, 127.4413876050234649 ) ;
#3594=ORIENTED_EDGE ( 'NONE', *, *, #745, .F. ) ;
#3598=CIRCLE ( 'NONE', #2256, 112.8770930172170637 ) ;
#3612=DIRECTION ( 'NONE',  ( -6.982962677686266711E-15, 0.000000000000000000, -1.000000000000000000 ) ) ;
#3618=CARTESIAN_POINT ( 'NONE',  ( -5.524863963826822655, -116.0870680293436408, 14.88498244535549020 ) ) ;
#3622=PRODUCT ( 'Vane Disc', 'Vane Disc', '', ( #17526 ) ) ;
#3626=ORIENTED_EDGE ( 'NONE', *, *, #8233, .F. ) ;
#3638=DIRECTION ( 'NONE',  ( 6.982962677686266711E-15, -0.000000000000000000, 1.000000000000000000 ) ) ;
#3656=CARTESIAN_POINT ( 'NONE',  ( 106.5208805777954524, 53.25886146954521649, 39.88498244535470860 ) ) ;
#3669=EDGE_LOOP ( 'NONE', ( #17242, #8196, #11928, #19491 ) ) ;
#3684=CYLINDRICAL_SURFACE ( 'NONE', #17994, 112.8770930172170210 ) ;
#3729=DIRECTION ( 'NONE',  ( 6.982962677686266711E-15, -0.000000000000000000, 1.000000000000000000 ) ) ;
#3757=CARTESIAN_POINT ( 'NONE',  ( 105.9946577255053626, 51.49356311920430329, 14.88498244535471215 ) ) ;
#3782=CYLINDRICAL_SURFACE ( 'NONE', #11661, 3.224098631618460331 ) ;
#3802=ADVANCED_FACE ( 'NONE', ( #14409 ), #390, .T. ) ;
#3811=ORIENTED_EDGE ( 'NONE', *, *, #14489, .T. ) ;
#3835=CIRCLE ( 'NONE', #7113, 112.8770930172170068 ) ;
#3863=CIRCLE ( 'NONE', #8760, 17.50000000000000355 ) ;
#3888=FACE_OUTER_BOUND ( 'NONE', #11057, .T. ) ;
#3890=EDGE_CURVE ( 'NONE', #16353, #8253, #724, .T. ) ;
#3899=EDGE_LOOP ( 'NONE', ( #9673, #1110, #17965, #14978 ) ) ;
#3905=EDGE_CURVE ( 'NONE', #19703, #6726, #12144, .T. ) ;
#3908=CIRCLE ( 'NONE', #12714, 112.8770930172170210 ) ;
#3912=CARTESIAN_POINT ( 'NONE',  ( -1.607844166819003129E-13, 26.82911281104372847, 14.88498244535545112 ) ) ;
#3939=CYLINDRICAL_SURFACE ( 'NONE', #429, 3.224098631618460331 ) ;
#3945=DIRECTION ( 'NONE',  ( -6.982962677686266711E-15, 0.000000000000000000, -1.000000000000000000 ) ) ;
#3954=DIRECTION ( 'NONE',  ( -0.7660444431189770143, 0.6427876096865405842, 5.348151281215662765E-15 ) ) ;
#3961=CARTESIAN_POINT ( 'NONE',  ( 14.85701326357424890, 22.71800723006102274, 39.88498244535534809 ) ) ;
#3964=EDGE_CURVE ( 'NONE', #15086, #15546, #10460, .T. ) ;
#3991=EDGE_CURVE ( 'NONE', #19110, #16155, #8565, .T. ) ;
#3998=DIRECTION ( 'NONE',  ( 0.9396926207859112035, 0.3420201433256609969, -6.456589605409174593E-15 ) ) ;
#4019=CARTESIAN_POINT ( 'NONE',  ( -14.69786621328411869, 22.52834316112731017, 14.88498244535555592 ) ) ;
#4024=ORIENTED_EDGE ( 'NONE', *, *, #19114, .T. ) ;
#4025=CARTESIAN_POINT ( 'NONE',  ( -26.42151830275515323, 4.658826548058537576, 14.88498244535563586 ) ) ;
#4036=ORIENTED_EDGE ( 'NONE', *, *, #8219, .F. ) ;
#4040=AXIS2_PLACEMENT_3D ( 'NONE', #15889, #17535, #19357 ) ;
#4058=VECTOR ( 'NONE', #19688, 1000.000000000000000 ) ;
#4087=CARTESIAN_POINT ( 'NONE',  ( -21.73104181959847025, -16.26654594725001957, 14.88498244535560389 ) ) ;
#4089=ORIENTED_EDGE ( 'NONE', *, *, #16386, .T. ) ;
#4101=DIRECTION ( 'NONE',  ( 6.982962677686266711E-15, -0.000000000000000000, 1.000000000000000000 ) ) ;
#4108=VERTEX_POINT ( 'NONE', #14055 ) ;
#4114=CARTESIAN_POINT ( 'NONE',  ( -97.77191798235051579, 62.82820655979934088, 14.88498244535613502 ) ) ;
#4125=CIRCLE ( 'NONE', #13924, 27.50000000000000355 ) ;
#4157=CARTESIAN_POINT ( 'NONE',  ( -23.23469325536255070, -13.41455640552162443, 39.88498244535561810 ) ) ;
#4162=ORIENTED_EDGE ( 'NONE', *, *, #14879, .F. ) ;
#4177=EDGE_LOOP ( 'NONE', ( #15426, #3594, #10500, #9250 ) ) ;
#4180=FACE_OUTER_BOUND ( 'NONE', #12731, .T. ) ;
#4200=LINE ( 'NONE', #18922, #13421 ) ;
#4207=FACE_OUTER_BOUND ( 'NONE', #11898, .T. ) ;
#4242=EDGE_CURVE ( 'NONE', #141, #19127, #11182, .T. ) ;
#4243=ORIENTED_EDGE ( 'NONE', *, *, #14284, .F. ) ;
#4252=CARTESIAN_POINT ( 'NONE',  ( 41.69438488732666315, 106.8146822993833780, 14.88498244535515980 ) ) ;
#4259=DIRECTION ( 'NONE',  ( -1.000000000000000000, 0.000000000000000000, 7.007922368489490773E-15 ) ) ;
#4281=CARTESIAN_POINT ( 'NONE',  ( 103.2967819461768073, 53.25886146954521649, 14.88498244535472992 ) ) ;
#4320=EDGE_CURVE ( 'NONE', #12923, #14390, #2682, .T. ) ;
#4321=ORIENTED_EDGE ( 'NONE', *, *, #5405, .F. ) ;
#4325=AXIS2_PLACEMENT_3D ( 'NONE', #15176, #6836, #14703 ) ;
#4332=AXIS2_PLACEMENT_3D ( 'NONE', #4487, #16973, #13893 ) ;
#4333=ORIENTED_EDGE ( 'NONE', *, *, #3119, .T. ) ;
#4336=ORIENTED_EDGE ( 'NONE', *, *, #3381, .F. ) ;
#4364=EDGE_CURVE ( 'NONE', #315, #17480, #5337, .T. ) ;
#4370=( LENGTH_UNIT ( ) NAMED_UNIT ( * ) SI_UNIT ( .MILLI., .METRE. ) );
#4376=EDGE_CURVE ( 'NONE', #16627, #3202, #10211, .T. ) ;
#4378=CYLINDRICAL_SURFACE ( 'NONE', #11392, 3.224098631618460331 ) ;
#4380=CARTESIAN_POINT ( 'NONE',  ( 25.98398601615827985, 7.853099154550822192, 14.88498244535527171 ) ) ;
#4382=DIRECTION ( 'NONE',  ( 6.982962677686266711E-15, -0.000000000000000000, 1.000000000000000000 ) ) ;
#4387=CARTESIAN_POINT ( 'NONE',  ( -63.98537287693023501, 94.20918150411493741, 39.88498244535590231 ) ) ;
#4397=CARTESIAN_POINT ( 'NONE',  ( -32.30548103355237544, 113.3261241031799926, 14.88498244535567672 ) ) ;
#4401=EDGE_CURVE ( 'NONE', #2341, #2918, #16758, .T. ) ;
#4406=DIRECTION ( 'NONE',  ( 1.000000000000000000, 0.000000000000000000, -6.994638739193269649E-15 ) ) ;
#4412=DIRECTION ( 'NONE',  ( 6.982962677686266711E-15, -0.000000000000000000, 1.000000000000000000 ) ) ;
#4423=DIRECTION ( 'NONE',  ( -6.982962677686266711E-15, 0.000000000000000000, -1.000000000000000000 ) ) ;
#4429=AXIS2_PLACEMENT_3D ( 'NONE', #16843, #19806, #2940 ) ;
#4450=EDGE_LOOP ( 'NONE', ( #16483, #11000, #14216, #15566, #17419 ) ) ;
#4472=CYLINDRICAL_SURFACE ( 'NONE', #582, 112.8770930172170210 ) ;
#4487=CARTESIAN_POINT ( 'NONE',  ( 11.54085525628735809, 113.2974248684783163, 39.88498244535537651 ) ) ;
#4497=ORIENTED_EDGE ( 'NONE', *, *, #14769, .F. ) ;
#4506=CARTESIAN_POINT ( 'NONE',  ( 11.54085525628735809, 113.2974248684783163, 39.88498244535537651 ) ) ;
#4514=LINE ( 'NONE', #1134, #7451 ) ;
#4522=ORIENTED_EDGE ( 'NONE', *, *, #2782, .F. ) ;
#4550=AXIS2_PLACEMENT_3D ( 'NONE', #13501, #18032, #10150 ) ;
#4562=DIRECTION ( 'NONE',  ( 0.9396926207859104263, 0.3420201433256629397, -6.456589605409169071E-15 ) ) ;
#4564=CARTESIAN_POINT ( 'NONE',  ( 73.61113626724137760, -92.47916748300480094, 39.88498244535494308 ) ) ;
#4568=AXIS2_PLACEMENT_3D ( 'NONE', #850, #2597, #17846 ) ;
#4580=( GEOMETRIC_REPRESENTATION_CONTEXT ( 3 ) GLOBAL_UNCERTAINTY_ASSIGNED_CONTEXT ( ( #7424 ) ) GLOBAL_UNIT_ASSIGNED_CONTEXT ( ( #13400, #2378, #643 ) ) REPRESENTATION_CONTEXT ( 'NONE', 'WORKASPACE' ) );
#4614=VERTEX_POINT ( 'NONE', #14340 ) ;
#4620=AXIS2_PLACEMENT_3D ( 'NONE', #17445, #11076, #9846 ) ;
#4651=ORIENTED_EDGE ( 'NONE', *, *, #19031, .F. ) ;
#4653=ADVANCED_FACE ( 'NONE', ( #11658 ), #5727, .T. ) ;
#4660=VECTOR ( 'NONE', #14509, 1000.000000000000000 ) ;
#4667=DIRECTION ( 'NONE',  ( 6.982962677686266711E-15, -0.000000000000000000, 1.000000000000000000 ) ) ;
#4705=ORIENTED_EDGE ( 'NONE', *, *, #18793, .F. ) ;
#4708=ORIENTED_EDGE ( 'NONE', *, *, #12218, .T. ) ;
#4716=FACE_OUTER_BOUND ( 'NONE', #6954, .T. ) ;
#4747=ADVANCED_FACE ( 'NONE', ( #13383 ), #14831, .F. ) ;
#4751=CYLINDRICAL_SURFACE ( 'NONE', #3194, 112.8770930172170210 ) ;
#4755=PRODUCT_DEFINITION_SHAPE ( 'NONE', 'NONE',  #8640 ) ;
#4758=ORIENTED_EDGE ( 'NONE', *, *, #12594, .F. ) ;
#4766=VECTOR ( 'NONE', #14523, 1000.000000000000000 ) ;
#4767=CARTESIAN_POINT ( 'NONE',  ( 27.90514497005392869, -110.4119590718113244, 39.88498244535525572 ) ) ;
#4770=CARTESIAN_POINT ( 'NONE',  ( 11.54085525628718401, 113.2974248684783163, 14.88498244535537296 ) ) ;
#4774=DIRECTION ( 'NONE',  ( -6.982962677686266711E-15, 0.000000000000000000, -1.000000000000000000 ) ) ;
#4783=ORIENTED_EDGE ( 'NONE', *, *, #10156, .F. ) ;
#4820=VERTEX_POINT ( 'NONE', #7453 ) ;
#4823=CARTESIAN_POINT ( 'NONE',  ( -23.19741967113669290, 4.658826548058537576, 14.88498244535561277 ) ) ;
#4842=DIRECTION ( 'NONE',  ( -6.982962677686266711E-15, 0.000000000000000000, -1.000000000000000000 ) ) ;
#4853=CYLINDRICAL_SURFACE ( 'NONE', #8676, 3.224098631618460331 ) ;
#4856=DIRECTION ( 'NONE',  ( 6.982962677686266711E-15, -0.000000000000000000, 1.000000000000000000 ) ) ;
#4869=EDGE_CURVE ( 'NONE', #9831, #18211, #9254, .T. ) ;
#4886=DIRECTION ( 'NONE',  ( -6.982962677686266711E-15, 0.000000000000000000, -1.000000000000000000 ) ) ;
#4887=ORIENTED_EDGE ( 'NONE', *, *, #17334, .F. ) ;
#4894=EDGE_CURVE ( 'NONE', #8253, #7528, #6336, .T. ) ;
#4908=CIRCLE ( 'NONE', #11420, 17.50000000000000355 ) ;
#4928=CARTESIAN_POINT ( 'NONE',  ( 70.38703763562291726, -92.47916748300480094, 39.88498244535495729 ) ) ;
#4935=LINE ( 'NONE', #6568, #18715 ) ;
#4941=DIRECTION ( 'NONE',  ( 1.000000000000000000, 0.000000000000000000, -6.977185866873308817E-15 ) ) ;
#4952=DIRECTION ( 'NONE',  ( 6.982962677686266711E-15, -0.000000000000000000, 1.000000000000000000 ) ) ;
#4961=CARTESIAN_POINT ( 'NONE',  ( -6.191009641800249597, -26.42934155884823255, 39.88498244535549730 ) ) ;
#4967=ORIENTED_EDGE ( 'NONE', *, *, #19795, .F. ) ;
#4992=DIRECTION ( 'NONE',  ( 6.982962677686266711E-15, -0.000000000000000000, 1.000000000000000000 ) ) ;
#5006=CARTESIAN_POINT ( 'NONE',  ( -23.23469325536272478, -13.41455640552162443, 14.88498244535561454 ) ) ;
#5028=DIRECTION ( 'NONE',  ( 1.000000000000000000, 0.000000000000000000, -6.994638739193269649E-15 ) ) ;
#5043=ORIENTED_EDGE ( 'NONE', *, *, #4376, .F. ) ;
#5047=CIRCLE ( 'NONE', #4040, 112.8770930172170210 ) ;
#5057=DIRECTION ( 'NONE',  ( -6.982962677686266711E-15, 0.000000000000000000, -1.000000000000000000 ) ) ;
#5067=CIRCLE ( 'NONE', #17474, 106.4288957539801004 ) ;
#5072=DIRECTION ( 'NONE',  ( -6.982962677686266711E-15, 7.888609052210118054E-31, -1.000000000000000000 ) ) ;
#5073=CARTESIAN_POINT ( 'NONE',  ( -63.98537287693041264, 94.20918150411493741, 14.88498244535589876 ) ) ;
#5075=DIRECTION ( 'NONE',  ( 0.4999999999999918954, -0.8660254037844431485, -3.520662956770156304E-15 ) ) ;
#5084=DIRECTION ( 'NONE',  ( 1.000000000000000000, 0.000000000000000000, -6.994638739193269649E-15 ) ) ;
#5086=CARTESIAN_POINT ( 'NONE',  ( 103.2967819461769921, 53.25886146954521649, 39.88498244535472992 ) ) ;
#5102=ORIENTED_EDGE ( 'NONE', *, *, #18991, .T. ) ;
#5105=CIRCLE ( 'NONE', #2171, 3.224098631618460331 ) ;
#5107=DIRECTION ( 'NONE',  ( -6.982962677686266711E-15, 0.000000000000000000, -1.000000000000000000 ) ) ;
#5129=VECTOR ( 'NONE', #2935, 1000.000000000000000 ) ;
#5156=EDGE_CURVE ( 'NONE', #7528, #20089, #8278, .T. ) ;
#5171=AXIS2_PLACEMENT_3D ( 'NONE', #11864, #16594, #2580 ) ;
#5185=ORIENTED_EDGE ( 'NONE', *, *, #12025, .T. ) ;
#5187=DIRECTION ( 'NONE',  ( -0.1736481776669280275, 0.9848077530122084644, 2.152196535136391663E-15 ) ) ;
#5213=AXIS2_PLACEMENT_3D ( 'NONE', #10660, #10451, #15374 ) ;
#5215=ORIENTED_EDGE ( 'NONE', *, *, #19520, .F. ) ;
#5221=FACE_OUTER_BOUND ( 'NONE', #15178, .T. ) ;
#5240=ORIENTED_EDGE ( 'NONE', *, *, #7603, .T. ) ;
#5254=CARTESIAN_POINT ( 'NONE',  ( -63.98537287693041264, 94.20918150411493741, 14.88498244535589876 ) ) ;
#5257=CARTESIAN_POINT ( 'NONE',  ( -27.10287801637868199, 1.507547295587424951, 14.88498244535564297 ) ) ;
#5267=CARTESIAN_POINT ( 'NONE',  ( 70.38703763562273252, -92.47916748300480094, 14.88498244535495907 ) ) ;
#5285=EDGE_CURVE ( 'NONE', #17930, #9086, #18482, .T. ) ;
#5294=CARTESIAN_POINT ( 'NONE',  ( 26.85905058935160383, 1.464553941565464035, 39.88498244535526283 ) ) ;
#5297=DIRECTION ( 'NONE',  ( -0.1736481776669280275, 0.9848077530122084644, 2.152196535136391663E-15 ) ) ;
#5302=EDGE_CURVE ( 'NONE', #16902, #7679, #2634, .T. ) ;
#5306=ORIENTED_EDGE ( 'NONE', *, *, #6535, .T. ) ;
#5333=EDGE_LOOP ( 'NONE', ( #1433, #15130, #11920, #17618 ) ) ;
#5337=CIRCLE ( 'NONE', #428, 106.4288957539801288 ) ;
#5338=AXIS2_PLACEMENT_3D ( 'NONE', #17679, #13724, #13048 ) ;
#5339=ORIENTED_EDGE ( 'NONE', *, *, #9253, .F. ) ;
#5358=EDGE_CURVE ( 'NONE', #2409, #8834, #10303, .T. ) ;
#5359=( GEOMETRIC_REPRESENTATION_CONTEXT ( 3 ) GLOBAL_UNCERTAINTY_ASSIGNED_CONTEXT ( ( #13552 ) ) GLOBAL_UNIT_ASSIGNED_CONTEXT ( ( #4370, #9071, #7539 ) ) REPRESENTATION_CONTEXT ( 'NONE', 'WORKASPACE' ) );
#5362=EDGE_CURVE ( 'NONE', #14667, #10450, #3459, .T. ) ;
#5363=DIRECTION ( 'NONE',  ( 0.9396926207859112035, 0.3420201433256609969, -6.456589605409174593E-15 ) ) ;
#5372=DIRECTION ( 'NONE',  ( -0.1736481776669408228, -0.9848077530122062440, 1.076098267568195042E-15 ) ) ;
#5374=DIRECTION ( 'NONE',  ( -6.982962677686266711E-15, 0.000000000000000000, -1.000000000000000000 ) ) ;
#5383=ORIENTED_EDGE ( 'NONE', *, *, #14484, .F. ) ;
#5396=DIRECTION ( 'NONE',  ( 6.982962677686266711E-15, -0.000000000000000000, 1.000000000000000000 ) ) ;
#5398=CARTESIAN_POINT ( 'NONE',  ( 91.98363426319514247, -42.08539992651071771, 14.88498244535480985 ) ) ;
#5403=DIRECTION ( 'NONE',  ( 1.000000000000000000, 0.000000000000000000, -6.994638739193269649E-15 ) ) ;
#5405=EDGE_CURVE ( 'NONE', #7679, #14667, #5105, .T. ) ;
#5426=CARTESIAN_POINT ( 'NONE',  ( 69.11703934647950121, -95.44259730872654757, 14.88498244535496973 ) ) ;
#5435=AXIS2_PLACEMENT_3D ( 'NONE', #10351, #1254, #10657 ) ;
#5444=DIRECTION ( 'NONE',  ( -0.1736481776669268895, 0.9848077530122086864, 2.152196535136390479E-15 ) ) ;
#5450=ORIENTED_EDGE ( 'NONE', *, *, #13991, .T. ) ;
#5463=CARTESIAN_POINT ( 'NONE',  ( -23.23469325536272478, -13.41455640552162443, 14.88498244535561454 ) ) ;
#5470=ORIENTED_EDGE ( 'NONE', *, *, #10225, .T. ) ;
#5472=SHAPE_REPRESENTATION ( 'Vane Disc', ( #18639 ), #4580 ) ;
#5473=CIRCLE ( 'NONE', #15924, 106.4288957539801146 ) ;
#5474=ORIENTED_EDGE ( 'NONE', *, *, #17363, .T. ) ;
#5497=DIRECTION ( 'NONE',  ( 0.4999999999999925060, -0.8660254037844429265, -3.228294802704592424E-15 ) ) ;
#5501=AXIS2_PLACEMENT_3D ( 'NONE', #11240, #9706, #12971 ) ;
#5506=ADVANCED_FACE ( 'NONE', ( #441 ), #4853, .T. ) ;
#5528=DIRECTION ( 'NONE',  ( 6.982962677686266711E-15, -0.000000000000000000, 1.000000000000000000 ) ) ;
#5548=DIRECTION ( 'NONE',  ( 6.982962677686266711E-15, -0.000000000000000000, 1.000000000000000000 ) ) ;
#5558=ORIENTED_EDGE ( 'NONE', *, *, #18687, .F. ) ;
#5582=ORIENTED_EDGE ( 'NONE', *, *, #15905, .T. ) ;
#5591=CARTESIAN_POINT ( 'NONE',  ( 48.09719419928496364, 107.5784105627835174, 14.88498244535511539 ) ) ;
#5592=AXIS2_PLACEMENT_3D ( 'NONE', #3618, #4856, #9648 ) ;
#5594=FACE_OUTER_BOUND ( 'NONE', #3425, .T. ) ;
#5603=EDGE_CURVE ( 'NONE', #295, #6917, #13231, .T. ) ;
#5604=ORIENTED_EDGE ( 'NONE', *, *, #15675, .T. ) ;
#5618=ORIENTED_EDGE ( 'NONE', *, *, #17150, .T. ) ;
#5619=CIRCLE ( 'NONE', #19029, 112.8770930172170210 ) ;
#5647=ORIENTED_EDGE ( 'NONE', *, *, #9199, .T. ) ;
#5648=DIRECTION ( 'NONE',  ( 6.982962677686266711E-15, -0.000000000000000000, 1.000000000000000000 ) ) ;
#5653=EDGE_LOOP ( 'NONE', ( #193, #4758, #14383, #11897 ) ) ;
#5698=DIRECTION ( 'NONE',  ( -6.982962677686266711E-15, 0.000000000000000000, -1.000000000000000000 ) ) ;
#5717=ADVANCED_FACE ( 'NONE', ( #9046 ), #7715, .T. ) ;
#5720=EDGE_LOOP ( 'NONE', ( #12365, #11062, #3445, #18934 ) ) ;
#5724=DIRECTION ( 'NONE',  ( -6.982962677686266711E-15, 0.000000000000000000, -1.000000000000000000 ) ) ;
#5726=FACE_OUTER_BOUND ( 'NONE', #7632, .T. ) ;
#5727=CYLINDRICAL_SURFACE ( 'NONE', #18402, 3.224098631618460331 ) ;
#5739=AXIS2_PLACEMENT_3D ( 'NONE', #9735, #4952, #538 ) ;
#5762=FACE_OUTER_BOUND ( 'NONE', #5720, .T. ) ;
#5774=CARTESIAN_POINT ( 'NONE',  ( 24.95276293194452322, -10.68636129284898573, 39.88498244535527704 ) ) ;
#5777=CARTESIAN_POINT ( 'NONE',  ( 44.89578954330598748, 107.1965464310834477, 39.88498244535514203 ) ) ;
#5782=EDGE_CURVE ( 'NONE', #2184, #2170, #17208, .T. ) ;
#5804=ORIENTED_EDGE ( 'NONE', *, *, #3125, .T. ) ;
#5805=DIRECTION ( 'NONE',  ( -1.000000000000000000, 0.000000000000000000, 6.976128451377903642E-15 ) ) ;
#5811=AXIS2_PLACEMENT_3D ( 'NONE', #3912, #5648, #5084 ) ;
#5825=ORIENTED_EDGE ( 'NONE', *, *, #11372, .T. ) ;
#5830=ORIENTED_EDGE ( 'NONE', *, *, #15675, .F. ) ;
#5844=DIRECTION ( 'NONE',  ( 6.982962677686266711E-15, -0.000000000000000000, 1.000000000000000000 ) ) ;
#5847=FACE_OUTER_BOUND ( 'NONE', #18651, .T. ) ;
#5850=CARTESIAN_POINT ( 'NONE',  ( 17.49999999999999289, 0.000000000000000000, 39.88498244535532677 ) ) ;
#5857=VECTOR ( 'NONE', #283, 1000.000000000000000 ) ;
#5861=EDGE_CURVE ( 'NONE', #11829, #2786, #19801, .T. ) ;
#5864=FACE_OUTER_BOUND ( 'NONE', #7305, .T. ) ;
#5865=CARTESIAN_POINT ( 'NONE',  ( 113.3640620605771261, -25.59923667990641150, 39.88498244535465886 ) ) ;
#5881=EDGE_CURVE ( 'NONE', #818, #6064, #15891, .T. ) ;
#5883=ORIENTED_EDGE ( 'NONE', *, *, #6897, .T. ) ;
#5891=ORIENTED_EDGE ( 'NONE', *, *, #16491, .T. ) ;
#5894=EDGE_LOOP ( 'NONE', ( #11916, #17425, #15032, #8904 ) ) ;
#5895=CARTESIAN_POINT ( 'NONE',  ( 21.51662357877997422, -16.14275151819498078, 14.88498244535530191 ) ) ;
#5907=CARTESIAN_POINT ( 'NONE',  ( 116.5881606921954017, -25.59923667990641150, 14.88498244535463755 ) ) ;
#5910=DIRECTION ( 'NONE',  ( 6.982962677686266711E-15, -0.000000000000000000, 1.000000000000000000 ) ) ;
#5921=CARTESIAN_POINT ( 'NONE',  ( -49.59485801383857506, -102.5175491340983882, 14.88498244535579929 ) ) ;
#5938=FACE_BOUND ( 'NONE', #18985, .T. ) ;
#5953=DIRECTION ( 'NONE',  ( -6.982962677686266711E-15, 0.000000000000000000, -1.000000000000000000 ) ) ;
#5981=ADVANCED_FACE ( 'NONE', ( #12707 ), #2156, .T. ) ;
#5986=ORIENTED_EDGE ( 'NONE', *, *, #12025, .F. ) ;
#5996=ORIENTED_EDGE ( 'NONE', *, *, #5285, .F. ) ;
#6008=ORIENTED_EDGE ( 'NONE', *, *, #3890, .F. ) ;
#6016=ORIENTED_EDGE ( 'NONE', *, *, #2665, .F. ) ;
#6052=ADVANCED_FACE ( 'NONE', ( #17708 ), #14146, .F. ) ;
#6056=DIRECTION ( 'NONE',  ( -6.982962677686266711E-15, -3.944304526105059027E-31, -1.000000000000000000 ) ) ;
#6059=DIRECTION ( 'NONE',  ( -1.000000000000000000, 0.000000000000000000, 6.456589605409171438E-15 ) ) ;
#6064=VERTEX_POINT ( 'NONE', #6183 ) ;
#6070=VERTEX_POINT ( 'NONE', #9547 ) ;
#6072=DIRECTION ( 'NONE',  ( -6.982962677686266711E-15, 0.000000000000000000, -1.000000000000000000 ) ) ;
#6101=CYLINDRICAL_SURFACE ( 'NONE', #16405, 106.4288957539801004 ) ;
#6114=VERTEX_POINT ( 'NONE', #8678 ) ;
#6139=DIRECTION ( 'NONE',  ( 0.5000000000000044409, 0.8660254037844360431, -3.228294802704586902E-15 ) ) ;
#6155=CARTESIAN_POINT ( 'NONE',  ( -26.42151830275497915, 4.658826548058537576, 39.88498244535563941 ) ) ;
#6157=ORIENTED_EDGE ( 'NONE', *, *, #4364, .F. ) ;
#6164=ORIENTED_EDGE ( 'NONE', *, *, #8028, .T. ) ;
#6183=CARTESIAN_POINT ( 'NONE',  ( 71.65703592476599226, -89.51573765728305432, 14.88498244535495196 ) ) ;
#6194=ORIENTED_EDGE ( 'NONE', *, *, #13642, .T. ) ;
#6195=AXIS2_PLACEMENT_3D ( 'NONE', #4025, #19385, #5372 ) ;
#6211=CARTESIAN_POINT ( 'NONE',  ( 92.34802049131684498, -66.64338626758360817, 14.88498244535480630 ) ) ;
#6212=DIRECTION ( 'NONE',  ( 6.982962677686266711E-15, -0.000000000000000000, 1.000000000000000000 ) ) ;
#6215=DIRECTION ( 'NONE',  ( -6.982962677686266711E-15, 0.000000000000000000, -1.000000000000000000 ) ) ;
#6223=VERTEX_POINT ( 'NONE', #16860 ) ;
#6232=DIRECTION ( 'NONE',  ( -0.1736481776669273613, 0.9848077530122085754, 1.206153050004590706E-15 ) ) ;
#6242=ORIENTED_EDGE ( 'NONE', *, *, #17738, .T. ) ;
#6247=AXIS2_PLACEMENT_3D ( 'NONE', #6612, #8133, #16222 ) ;
#6264=CARTESIAN_POINT ( 'NONE',  ( -97.77191798235051579, 62.82820655979934088, 14.88498244535613502 ) ) ;
#6273=VERTEX_POINT ( 'NONE', #16965 ) ;
#6288=CARTESIAN_POINT ( 'NONE',  ( 27.90514497005375461, -110.4119590718113244, 14.88498244535525750 ) ) ;
#6297=CIRCLE ( 'NONE', #9205, 112.8770930172170495 ) ;
#6300=EDGE_LOOP ( 'NONE', ( #12339, #4522, #7710, #14563 ) ) ;
#6310=CARTESIAN_POINT ( 'NONE',  ( -109.5721339228237667, 31.03941509555038181, 14.88498244535621851 ) ) ;
#6329=LINE ( 'NONE', #9589, #2212 ) ;
#6331=CARTESIAN_POINT ( 'NONE',  ( 3.221721112346448201, 26.70531838198836283, 39.88498244535543336 ) ) ;
#6336=CIRCLE ( 'NONE', #10552, 112.8770930172170637 ) ;
#6337=CARTESIAN_POINT ( 'NONE',  ( -2.647132857508548209, -114.6332882433608376, 14.88498244535546888 ) ) ;
#6342=EDGE_LOOP ( 'NONE', ( #12963, #9955, #16291, #863 ) ) ;
#6350=CYLINDRICAL_SURFACE ( 'NONE', #9266, 112.8770930172170068 ) ;
#6357=CARTESIAN_POINT ( 'NONE',  ( 114.2960429025576587, -28.68569479505797659, 14.88498244535465354 ) ) ;
#6377=DIRECTION ( 'NONE',  ( -1.000000000000000000, 0.000000000000000000, 6.969309079188926949E-15 ) ) ;
#6404=CARTESIAN_POINT ( 'NONE',  ( 19.63382932406824466, 18.38657833536341357, 14.88498244535531256 ) ) ;
#6408=CARTESIAN_POINT ( 'NONE',  ( -24.73834469112680523, -10.56256686379325593, 39.88498244535562520 ) ) ;
#6415=EDGE_CURVE ( 'NONE', #13679, #6070, #18168, .T. ) ;
#6439=CARTESIAN_POINT ( 'NONE',  ( -8.402595070144922573, -117.5408478153264298, 39.88498244535551862 ) ) ;
#6452=VERTEX_POINT ( 'NONE', #8458 ) ;
#6492=DIRECTION ( 'NONE',  ( -6.982962677686266711E-15, 0.000000000000000000, -1.000000000000000000 ) ) ;
#6502=ORIENTED_EDGE ( 'NONE', *, *, #5861, .F. ) ;
#6511=ADVANCED_FACE ( 'NONE', ( #10377 ), #11714, .F. ) ;
#6524=ORIENTED_EDGE ( 'NONE', *, *, #8233, .T. ) ;
#6534=ORIENTED_EDGE ( 'NONE', *, *, #11874, .F. ) ;
#6535=EDGE_CURVE ( 'NONE', #7331, #20085, #2195, .T. ) ;
#6539=ORIENTED_EDGE ( 'NONE', *, *, #19103, .T. ) ;
#6552=ORIENTED_EDGE ( 'NONE', *, *, #15997, .T. ) ;
#6555=AXIS2_PLACEMENT_3D ( 'NONE', #17638, #3612, #9842 ) ;
#6560=LINE ( 'NONE', #13072, #4766 ) ;
#6561=DIRECTION ( 'NONE',  ( 6.982962677686266711E-15, -0.000000000000000000, 1.000000000000000000 ) ) ;
#6568=CARTESIAN_POINT ( 'NONE',  ( -97.95177330934026827, 59.60912842347561025, 14.88498244535613502 ) ) ;
#6612=CARTESIAN_POINT ( 'NONE',  ( 1.396592535537253342E-14, 0.000000000000000000, 43.88498244535545467 ) ) ;
#6618=EDGE_CURVE ( 'NONE', #8834, #818, #227, .T. ) ;
#6628=DIRECTION ( 'NONE',  ( 1.000000000000000000, 0.000000000000000000, -7.137148015447434001E-15 ) ) ;
#6669=LINE ( 'NONE', #1748, #1874 ) ;
#6683=ADVANCED_FACE ( 'NONE', ( #20103 ), #6101, .F. ) ;
#6685=ORIENTED_EDGE ( 'NONE', *, *, #12462, .F. ) ;
#6710=LINE ( 'NONE', #12527, #12145 ) ;
#6721=EDGE_CURVE ( 'NONE', #10957, #18684, #17460, .T. ) ;
#6726=VERTEX_POINT ( 'NONE', #6408 ) ;
#6729=DIRECTION ( 'NONE',  ( 1.000000000000000000, 0.000000000000000000, -6.994638739193269649E-15 ) ) ;
#6731=EDGE_CURVE ( 'NONE', #20085, #7290, #11169, .T. ) ;
#6734=CARTESIAN_POINT ( 'NONE',  ( -17.24542129382105315, 20.55229278271246329, 39.88498244535557546 ) ) ;
#6744=VERTEX_POINT ( 'NONE', #7923 ) ;
#6760=EDGE_CURVE ( 'NONE', #19007, #11829, #6297, .T. ) ;
#6769=CIRCLE ( 'NONE', #2506, 3.224098631618459443 ) ;
#6792=DIRECTION ( 'NONE',  ( 6.982962677686266711E-15, -0.000000000000000000, 1.000000000000000000 ) ) ;
#6795=CARTESIAN_POINT ( 'NONE',  ( 81.66698895276897474, 79.37254397626031732, 39.88498244535488624 ) ) ;
#6817=ORIENTED_EDGE ( 'NONE', *, *, #15413, .F. ) ;
#6833=DIRECTION ( 'NONE',  ( 0.9396926207859104263, 0.3420201433256630508, -6.561838499445206374E-15 ) ) ;
#6836=DIRECTION ( 'NONE',  ( -6.982962677686266711E-15, 0.000000000000000000, -1.000000000000000000 ) ) ;
#6843=ORIENTED_EDGE ( 'NONE', *, *, #15595, .T. ) ;
#6856=DIRECTION ( 'NONE',  ( 0.9396926207859058744, -0.3420201433256757073, -6.562243095054852012E-15 ) ) ;
#6857=EDGE_CURVE ( 'NONE', #6064, #7509, #6710, .T. ) ;
#6870=ADVANCED_FACE ( 'NONE', ( #9865 ), #18787, .T. ) ;
#6885=CARTESIAN_POINT ( 'NONE',  ( -5.951998377315654842, -25.21111933077039069, 14.88498244535549198 ) ) ;
#6886=CYLINDRICAL_SURFACE ( 'NONE', #15431, 3.224098631618460331 ) ;
#6890=EDGE_LOOP ( 'NONE', ( #5185, #17513, #19459, #12904 ) ) ;
#6893=ORIENTED_EDGE ( 'NONE', *, *, #19551, .T. ) ;
#6897=EDGE_CURVE ( 'NONE', #6948, #6452, #5619, .T. ) ;
#6917=VERTEX_POINT ( 'NONE', #8435 ) ;
#6930=CARTESIAN_POINT ( 'NONE',  ( -97.59206265536077751, 66.04728469612305730, 14.88498244535613146 ) ) ;
#6931=DIRECTION ( 'NONE',  ( 6.982962677686266711E-15, -0.000000000000000000, 1.000000000000000000 ) ) ;
#6934=DIRECTION ( 'NONE',  ( -6.982962677686266711E-15, 0.000000000000000000, -1.000000000000000000 ) ) ;
#6936=CARTESIAN_POINT ( 'NONE',  ( 113.3640620605769413, -25.59923667990641150, 14.88498244535466064 ) ) ;
#6939=VECTOR ( 'NONE', #1694, 1000.000000000000000 ) ;
#6948=VERTEX_POINT ( 'NONE', #10453 ) ;
#6954=EDGE_LOOP ( 'NONE', ( #14416, #9655, #5830, #15409 ) ) ;
#6961=CARTESIAN_POINT ( 'NONE',  ( 97.51552550667287278, 26.88665364817694581, 14.88498244535477255 ) ) ;
#6970=EDGE_LOOP ( 'NONE', ( #7535, #9582, #19376, #17099 ) ) ;
#6984=CYLINDRICAL_SURFACE ( 'NONE', #2917, 27.50000000000000355 ) ;
#6985=DIRECTION ( 'NONE',  ( 6.982962677686266711E-15, -0.000000000000000000, 1.000000000000000000 ) ) ;
#6998=AXIS2_PLACEMENT_3D ( 'NONE', #14141, #6072, #10963 ) ;
#7018=EDGE_CURVE ( 'NONE', #19110, #16400, #18975, .T. ) ;
#7019=EDGE_LOOP ( 'NONE', ( #4887, #4705, #8064, #5986, #1839, #6534 ) ) ;
#7038=VERTEX_POINT ( 'NONE', #1676 ) ;
#7043=AXIS2_PLACEMENT_3D ( 'NONE', #19435, #9814, #10116 ) ;
#7047=CARTESIAN_POINT ( 'NONE',  ( 48.09719419928496364, 107.5784105627835174, 14.88498244535511539 ) ) ;
#7059=FACE_OUTER_BOUND ( 'NONE', #3196, .T. ) ;
#7088=LINE ( 'NONE', #18035, #11684 ) ;
#7096=CYLINDRICAL_SURFACE ( 'NONE', #451, 3.224098631618460331 ) ;
#7102=DIRECTION ( 'NONE',  ( -1.000000000000000000, 0.000000000000000000, 6.456589605409171438E-15 ) ) ;
#7106=DIRECTION ( 'NONE',  ( 6.982962677686266711E-15, 0.000000000000000000, 1.000000000000000000 ) ) ;
#7111=CIRCLE ( 'NONE', #3191, 3.224098631618459443 ) ;
#7113=AXIS2_PLACEMENT_3D ( 'NONE', #17464, #15919, #1900 ) ;
#7119=DIRECTION ( 'NONE',  ( 6.982962677686266711E-15, -0.000000000000000000, 1.000000000000000000 ) ) ;
#7129=DIRECTION ( 'NONE',  ( 6.982962677686266711E-15, -0.000000000000000000, 1.000000000000000000 ) ) ;
#7132=ADVANCED_FACE ( 'NONE', ( #2287 ), #6886, .T. ) ;
#7185=CIRCLE ( 'NONE', #5501, 106.4288957539801146 ) ;
#7186=LINE ( 'NONE', #5850, #12821 ) ;
#7203=CARTESIAN_POINT ( 'NONE',  ( -34.51244174799973763, 110.9757759606085017, 39.88498244535569626 ) ) ;
#7209=VECTOR ( 'NONE', #8583, 1000.000000000000000 ) ;
#7219=AXIS2_PLACEMENT_3D ( 'NONE', #18452, #12199, #12408 ) ;
#7222=ORIENTED_EDGE ( 'NONE', *, *, #4894, .T. ) ;
#7241=DIRECTION ( 'NONE',  ( 0.9396926207859057634, -0.3420201433256758183, -6.456589605409169860E-15 ) ) ;
#7243=CARTESIAN_POINT ( 'NONE',  ( 27.90514497005375461, -110.4119590718113244, 14.88498244535525750 ) ) ;
#7250=VERTEX_POINT ( 'NONE', #931 ) ;
#7263=FACE_OUTER_BOUND ( 'NONE', #16751, .T. ) ;
#7264=ADVANCED_FACE ( 'NONE', ( #12379 ), #19849, .T. ) ;
#7275=DIRECTION ( 'NONE',  ( -6.982962677686266711E-15, 0.000000000000000000, -1.000000000000000000 ) ) ;
#7284=ADVANCED_FACE ( 'NONE', ( #5847 ), #7469, .F. ) ;
#7290=VERTEX_POINT ( 'NONE', #19950 ) ;
#7298=CIRCLE ( 'NONE', #11553, 3.224098631618458999 ) ;
#7305=EDGE_LOOP ( 'NONE', ( #16444, #9480, #14567, #14590 ) ) ;
#7308=ORIENTED_EDGE ( 'NONE', *, *, #19114, .F. ) ;
#7316=ORIENTED_EDGE ( 'NONE', *, *, #7762, .F. ) ;
#7324=ORIENTED_EDGE ( 'NONE', *, *, #17180, .F. ) ;
#7331=VERTEX_POINT ( 'NONE', #2676 ) ;
#7335=ADVANCED_FACE ( 'NONE', ( #18430 ), #1340, .T. ) ;
#7338=VECTOR ( 'NONE', #10922, 1000.000000000000000 ) ;
#7351=ORIENTED_EDGE ( 'NONE', *, *, #19509, .F. ) ;
#7354=DIRECTION ( 'NONE',  ( -0.7660444431189770143, 0.6427876096865404731, 5.348151281215661977E-15 ) ) ;
#7366=EDGE_CURVE ( 'NONE', #2014, #13413, #16995, .T. ) ;
#7367=DIRECTION ( 'NONE',  ( -0.1736481776669273613, 0.9848077530122085754, 1.238751781085795780E-15 ) ) ;
#7369=DIRECTION ( 'NONE',  ( 6.982962677686266711E-15, -0.000000000000000000, 1.000000000000000000 ) ) ;
#7417=ORIENTED_EDGE ( 'NONE', *, *, #17876, .T. ) ;
#7422=AXIS2_PLACEMENT_3D ( 'NONE', #2593, #18236, #16806 ) ;
#7424=UNCERTAINTY_MEASURE_WITH_UNIT (LENGTH_MEASURE( 1.000000000000000082E-05 ), #13400, 'distance_accuracy_value', 'NONE');
#7432=ORIENTED_EDGE ( 'NONE', *, *, #19795, .T. ) ;
#7440=DIRECTION ( 'NONE',  ( 1.000000000000000000, 0.000000000000000000, 0.000000000000000000 ) ) ;
#7451=VECTOR ( 'NONE', #9007, 1000.000000000000000 ) ;
#7452=FACE_BOUND ( 'NONE', #7583, .T. ) ;
#7453=CARTESIAN_POINT ( 'NONE',  ( -12.16118437606760949, -23.99289710269258080, 39.88498244535554704 ) ) ;
#7458=DIRECTION ( 'NONE',  ( 0.5000000000000039968, 0.8660254037844362651, -3.488592933436653225E-15 ) ) ;
#7469=CYLINDRICAL_SURFACE ( 'NONE', #14784, 106.4288957539800862 ) ;
#7473=ORIENTED_EDGE ( 'NONE', *, *, #3002, .F. ) ;
#7477=EDGE_CURVE ( 'NONE', #17480, #17433, #18638, .T. ) ;
#7478=ORIENTED_EDGE ( 'NONE', *, *, #3119, .F. ) ;
#7482=ORIENTED_EDGE ( 'NONE', *, *, #14262, .T. ) ;
#7507=VECTOR ( 'NONE', #19360, 1000.000000000000000 ) ;
#7509=VERTEX_POINT ( 'NONE', #18950 ) ;
#7511=EDGE_CURVE ( 'NONE', #17939, #7290, #4935, .T. ) ;
#7523=CARTESIAN_POINT ( 'NONE',  ( -17.24542129382122724, 20.55229278271246329, 14.88498244535557369 ) ) ;
#7528=VERTEX_POINT ( 'NONE', #8489 ) ;
#7532=ORIENTED_EDGE ( 'NONE', *, *, #1371, .T. ) ;
#7535=ORIENTED_EDGE ( 'NONE', *, *, #904, .F. ) ;
#7536=EDGE_LOOP ( 'NONE', ( #8993, #20092 ) ) ;
#7539=( NAMED_UNIT ( * ) SI_UNIT ( $, .STERADIAN. ) SOLID_ANGLE_UNIT ( ) );
#7541=ORIENTED_EDGE ( 'NONE', *, *, #16801, .F. ) ;
#7583=EDGE_LOOP ( 'NONE', ( #17913, #10366, #16331, #15853, #6502 ) ) ;
#7585=DIRECTION ( 'NONE',  ( -1.000000000000000000, 0.000000000000000000, 7.065055611250995019E-15 ) ) ;
#7603=EDGE_CURVE ( 'NONE', #2409, #6948, #8586, .T. ) ;
#7628=ADVANCED_FACE ( 'NONE', ( #7059 ), #9925, .T. ) ;
#7632=EDGE_LOOP ( 'NONE', ( #1235, #1308, #2670, #4333, #12869 ) ) ;
#7640=ORIENTED_EDGE ( 'NONE', *, *, #3991, .F. ) ;
#7648=CIRCLE ( 'NONE', #8311, 3.224098631618458999 ) ;
#7652=CYLINDRICAL_SURFACE ( 'NONE', #10052, 3.224098631618460331 ) ;
#7656=FACE_BOUND ( 'NONE', #18254, .T. ) ;
#7668=ADVANCED_FACE ( 'NONE', ( #12648 ), #18908, .F. ) ;
#7679=VERTEX_POINT ( 'NONE', #9684 ) ;
#7683=EDGE_LOOP ( 'NONE', ( #3477, #17134, #6817, #13691 ) ) ;
#7710=ORIENTED_EDGE ( 'NONE', *, *, #6618, .F. ) ;
#7715=CYLINDRICAL_SURFACE ( 'NONE', #11943, 27.50000000000000355 ) ;
#7744=CARTESIAN_POINT ( 'NONE',  ( 11.54085525628718401, 113.2974248684783163, 14.88498244535537296 ) ) ;
#7761=AXIS2_PLACEMENT_3D ( 'NONE', #15632, #11116, #2023 ) ;
#7762=EDGE_CURVE ( 'NONE', #2440, #17104, #1060, .T. ) ;
#7778=CARTESIAN_POINT ( 'NONE',  ( 112.4320812185962524, -22.51277856475483574, 14.88498244535466775 ) ) ;
#7795=ADVANCED_FACE ( 'NONE', ( #5864 ), #3939, .T. ) ;
#7804=CARTESIAN_POINT ( 'NONE',  ( 81.66698895276879000, 79.37254397626031732, 14.88498244535488269 ) ) ;
#7809=DIRECTION ( 'NONE',  ( 6.982962677686266711E-15, -0.000000000000000000, 1.000000000000000000 ) ) ;
#7834=EDGE_LOOP ( 'NONE', ( #1698, #14973, #16189, #17820, #4651 ) ) ;
#7864=VERTEX_POINT ( 'NONE', #8000 ) ;
#7922=CARTESIAN_POINT ( 'NONE',  ( -17.24542129382122724, 20.55229278271246329, 14.88498244535557369 ) ) ;
#7923=CARTESIAN_POINT ( 'NONE',  ( 17.49999999999999289, 0.000000000000000000, 39.88498244535532677 ) ) ;
#7939=VERTEX_POINT ( 'NONE', #18544 ) ;
#7957=DIRECTION ( 'NONE',  ( 6.982962677686266711E-15, -0.000000000000000000, 1.000000000000000000 ) ) ;
#8000=CARTESIAN_POINT ( 'NONE',  ( 106.5208805777952676, 53.25886146954521649, 14.88498244535470683 ) ) ;
#8028=EDGE_CURVE ( 'NONE', #9259, #807, #18966, .T. ) ;
#8029=CARTESIAN_POINT ( 'NONE',  ( -103.8888757476051836, -46.65403860089418941, 39.88498244535617943 ) ) ;
#8031=CARTESIAN_POINT ( 'NONE',  ( -81.99056186900656940, -84.64042930812179577, 39.88498244535603021 ) ) ;
#8058=CIRCLE ( 'NONE', #3480, 3.224098631618459443 ) ;
#8064=ORIENTED_EDGE ( 'NONE', *, *, #12348, .F. ) ;
#8085=CARTESIAN_POINT ( 'NONE',  ( -109.5721339228235820, 31.03941509555038181, 39.88498244535622206 ) ) ;
#8088=EDGE_LOOP ( 'NONE', ( #9456, #15028, #1830, #11918 ) ) ;
#8092=ORIENTED_EDGE ( 'NONE', *, *, #5362, .F. ) ;
#8093=ADVANCED_FACE ( 'NONE', ( #8304 ), #14551, .T. ) ;
#8109=CARTESIAN_POINT ( 'NONE',  ( 127.4413876050234364, 0.000000000000000000, 39.88498244535456649 ) ) ;
#8115=CIRCLE ( 'NONE', #1244, 27.50000000000000355 ) ;
#8119=EDGE_LOOP ( 'NONE', ( #1600, #16488, #9329, #20196 ) ) ;
#8126=AXIS2_PLACEMENT_3D ( 'NONE', #12957, #11527, #9995 ) ;
#8131=DIRECTION ( 'NONE',  ( 6.982962677686266711E-15, -0.000000000000000000, 1.000000000000000000 ) ) ;
#8133=DIRECTION ( 'NONE',  ( -6.982962677686266711E-15, 0.000000000000000000, -1.000000000000000000 ) ) ;
#8161=AXIS2_PLACEMENT_3D ( 'NONE', #18209, #16581, #7458 ) ;
#8173=CARTESIAN_POINT ( 'NONE',  ( -14.02132266220276691, 20.55229278271246329, 14.88498244535555060 ) ) ;
#8176=CIRCLE ( 'NONE', #1980, 106.4288957539801004 ) ;
#8177=DIRECTION ( 'NONE',  ( 0.000000000000000000, 0.000000000000000000, 1.000000000000000000 ) ) ;
#8184=DIRECTION ( 'NONE',  ( 0.4999999999999919509, -0.8660254037844432595, -3.488592933436654014E-15 ) ) ;
#8194=EDGE_LOOP ( 'NONE', ( #13403, #13131 ) ) ;
#8196=ORIENTED_EDGE ( 'NONE', *, *, #6857, .F. ) ;
#8219=EDGE_CURVE ( 'NONE', #19500, #6948, #19140, .T. ) ;
#8220=ORIENTED_EDGE ( 'NONE', *, *, #2499, .F. ) ;
#8233=EDGE_CURVE ( 'NONE', #2918, #7528, #6560, .T. ) ;
#8250=AXIS2_PLACEMENT_3D ( 'NONE', #13277, #5724, #11840 ) ;
#8253=VERTEX_POINT ( 'NONE', #14716 ) ;
#8263=CARTESIAN_POINT ( 'NONE',  ( -6.191009641800430785, -26.42934155884822900, 14.88498244535549375 ) ) ;
#8277=CARTESIAN_POINT ( 'NONE',  ( 27.50000000000001776, 3.367778697655222096E-15, 127.7817459305202448 ) ) ;
#8278=CIRCLE ( 'NONE', #2086, 112.8770930172170637 ) ;
#8291=DIRECTION ( 'NONE',  ( 6.982962677686266711E-15, -0.000000000000000000, 1.000000000000000000 ) ) ;
#8295=ORIENTED_EDGE ( 'NONE', *, *, #11291, .F. ) ;
#8304=FACE_OUTER_BOUND ( 'NONE', #19158, .T. ) ;
#8311=AXIS2_PLACEMENT_3D ( 'NONE', #17092, #1648, #17202 ) ;
#8329=CARTESIAN_POINT ( 'NONE',  ( -3.221721112346616067, 26.95290724009910832, 14.88498244535547244 ) ) ;
#8332=VECTOR ( 'NONE', #11827, 1000.000000000000000 ) ;
#8337=ORIENTED_EDGE ( 'NONE', *, *, #745, .T. ) ;
#8340=ORIENTED_EDGE ( 'NONE', *, *, #6415, .T. ) ;
#8345=ADVANCED_FACE ( 'NONE', ( #996 ), #10115, .T. ) ;
#8352=LINE ( 'NONE', #9689, #5857 ) ;
#8380=DIRECTION ( 'NONE',  ( 6.982962677686266711E-15, -0.000000000000000000, 1.000000000000000000 ) ) ;
#8416=CARTESIAN_POINT ( 'NONE',  ( 0.000000000000000000, 0.000000000000000000, 0.000000000000000000 ) ) ;
#8424=AXIS2_PLACEMENT_3D ( 'NONE', #10913, #379, #9491 ) ;
#8426=CIRCLE ( 'NONE', #5171, 3.224098631618460331 ) ;
#8435=CARTESIAN_POINT ( 'NONE',  ( 127.4413876050234933, 0.000000000000000000, 43.88498244535456649 ) ) ;
#8437=CYLINDRICAL_SURFACE ( 'NONE', #3322, 3.224098631618460331 ) ;
#8443=ORIENTED_EDGE ( 'NONE', *, *, #17420, .T. ) ;
#8458=CARTESIAN_POINT ( 'NONE',  ( 6.106329265062965028, -26.19668413589285194, 39.88498244535541204 ) ) ;
#8465=AXIS2_PLACEMENT_3D ( 'NONE', #5398, #14504, #6833 ) ;
#8482=EDGE_CURVE ( 'NONE', #19127, #19558, #9010, .T. ) ;
#8489=CARTESIAN_POINT ( 'NONE',  ( 48.89172014028676472, 94.20918150411493741, 39.88498244535511361 ) ) ;
#8494=ADVANCED_FACE ( 'NONE', ( #17067 ), #3056, .T. ) ;
#8500=CARTESIAN_POINT ( 'NONE',  ( 11.54085525628718401, 113.2974248684783163, 14.88498244535537296 ) ) ;
#8511=AXIS2_PLACEMENT_3D ( 'NONE', #89, #19122, #15541 ) ;
#8514=DIRECTION ( 'NONE',  ( -0.7660444431189770143, 0.6427876096865404731, 5.346191897317644801E-15 ) ) ;
#8522=DIRECTION ( 'NONE',  ( 6.982962677686266711E-15, -0.000000000000000000, 1.000000000000000000 ) ) ;
#8547=VERTEX_POINT ( 'NONE', #3656 ) ;
#8561=CARTESIAN_POINT ( 'NONE',  ( 27.90514497005392869, -110.4119590718113244, 39.88498244535525572 ) ) ;
#8565=CIRCLE ( 'NONE', #4325, 3.224098631618461219 ) ;
#8566=AXIS2_PLACEMENT_3D ( 'NONE', #8029, #3230, #11304 ) ;
#8577=EDGE_CURVE ( 'NONE', #912, #2426, #14576, .T. ) ;
#8583=DIRECTION ( 'NONE',  ( 6.982962677686266711E-15, -0.000000000000000000, 1.000000000000000000 ) ) ;
#8586=LINE ( 'NONE', #5426, #16113 ) ;
#8591=VERTEX_POINT ( 'NONE', #6331 ) ;
#8617=DIRECTION ( 'NONE',  ( -0.7660444431189862291, -0.6427876096865298150, 5.380491337840976593E-15 ) ) ;
#8629=AXIS2_PLACEMENT_3D ( 'NONE', #11959, #8805, #3998 ) ;
#8636=DIRECTION ( 'NONE',  ( 0.9396926207859104263, 0.3420201433256630508, -6.584943678403439596E-15 ) ) ;
#8640=PRODUCT_DEFINITION ( 'UNKNOWN', '', #12075, #13124 ) ;
#8643=CIRCLE ( 'NONE', #11882, 3.224098631618455890 ) ;
#8645=EDGE_LOOP ( 'NONE', ( #16583, #18903, #15023, #14554 ) ) ;
#8676=AXIS2_PLACEMENT_3D ( 'NONE', #334, #11282, #9742 ) ;
#8678=CARTESIAN_POINT ( 'NONE',  ( 14.85701326357409968, 22.71800723006099432, 14.88498244535534809 ) ) ;
#8701=CARTESIAN_POINT ( 'NONE',  ( 6.106329265062790945, -26.19668413589285194, 14.88498244535541026 ) ) ;
#8714=EDGE_CURVE ( 'NONE', #17576, #1080, #15216, .T. ) ;
#8716=EDGE_LOOP ( 'NONE', ( #10375, #18183, #10740, #14418, #10651, #6539 ) ) ;
#8730=DIRECTION ( 'NONE',  ( 0.5000000000000044409, 0.8660254037844360431, -4.304393070272782536E-15 ) ) ;
#8731=CARTESIAN_POINT ( 'NONE',  ( 12.24586475280392506, -24.22555452564823497, 14.88498244535536585 ) ) ;
#8760=AXIS2_PLACEMENT_3D ( 'NONE', #1946, #8177, #19131 ) ;
#8783=FACE_OUTER_BOUND ( 'NONE', #13717, .T. ) ;
#8805=DIRECTION ( 'NONE',  ( -6.982962677686266711E-15, 0.000000000000000000, -1.000000000000000000 ) ) ;
#8806=CARTESIAN_POINT ( 'NONE',  ( -25.47323767126238181, -97.89424917625660783, 14.88498244535562876 ) ) ;
#8809=AXIS2_PLACEMENT_3D ( 'NONE', #5463, #13218, #19480 ) ;
#8812=DIRECTION ( 'NONE',  ( 6.982962677686266711E-15, 0.000000000000000000, 1.000000000000000000 ) ) ;
#8814=ORIENTED_EDGE ( 'NONE', *, *, #15257, .F. ) ;
#8834=VERTEX_POINT ( 'NONE', #8701 ) ;
#8839=EDGE_CURVE ( 'NONE', #1401, #19110, #12564, .T. ) ;
#8852=CARTESIAN_POINT ( 'NONE',  ( -17.50000000000001776, 2.143131898507868643E-15, 39.88498244535557546 ) ) ;
#8856=DIRECTION ( 'NONE',  ( 1.000000000000000000, 0.000000000000000000, 0.000000000000000000 ) ) ;
#8859=CARTESIAN_POINT ( 'NONE',  ( -36.71940246244744799, 108.6254278180370250, 14.88498244535570869 ) ) ;
#8868=DIRECTION ( 'NONE',  ( -6.982962677686266711E-15, 0.000000000000000000, -1.000000000000000000 ) ) ;
#8888=EDGE_CURVE ( 'NONE', #1501, #10728, #306, .T. ) ;
#8892=DIRECTION ( 'NONE',  ( 6.982962677686266711E-15, -0.000000000000000000, 1.000000000000000000 ) ) ;
#8904=ORIENTED_EDGE ( 'NONE', *, *, #8888, .T. ) ;
#8906=CARTESIAN_POINT ( 'NONE',  ( 81.66698895276879000, 79.37254397626031732, 14.88498244535488269 ) ) ;
#8939=AXIS2_PLACEMENT_3D ( 'NONE', #10431, #15143, #2286 ) ;
#8959=CARTESIAN_POINT ( 'NONE',  ( -109.5721339228237667, 31.03941509555038181, 14.88498244535621851 ) ) ;
#8969=CARTESIAN_POINT ( 'NONE',  ( -23.19741967113669290, 4.658826548058537576, 14.88498244535561277 ) ) ;
#8977=ORIENTED_EDGE ( 'NONE', *, *, #14138, .T. ) ;
#8989=ORIENTED_EDGE ( 'NONE', *, *, #12218, .F. ) ;
#8993=ORIENTED_EDGE ( 'NONE', *, *, #13003, .F. ) ;
#9002=DIRECTION ( 'NONE',  ( 0.4999999999999919509, -0.8660254037844432595, -3.491481338843076952E-15 ) ) ;
#9004=LINE ( 'NONE', #15245, #18259 ) ;
#9007=DIRECTION ( 'NONE',  ( 6.982962677686266711E-15, -0.000000000000000000, 1.000000000000000000 ) ) ;
#9010=CIRCLE ( 'NONE', #19444, 106.4288957539801004 ) ;
#9029=AXIS2_PLACEMENT_3D ( 'NONE', #19197, #4886, #17365 ) ;
#9041=ORIENTED_EDGE ( 'NONE', *, *, #904, .T. ) ;
#9042=DIRECTION ( 'NONE',  ( -6.982962677686266711E-15, 0.000000000000000000, -1.000000000000000000 ) ) ;
#9046=FACE_OUTER_BOUND ( 'NONE', #6970, .T. ) ;
#9049=LINE ( 'NONE', #5895, #17612 ) ;
#9054=AXIS2_PLACEMENT_3D ( 'NONE', #14921, #908, #14531 ) ;
#9058=CARTESIAN_POINT ( 'NONE',  ( 41.69438488732684078, 106.8146822993833780, 39.88498244535516335 ) ) ;
#9071=( NAMED_UNIT ( * ) PLANE_ANGLE_UNIT ( ) SI_UNIT ( $, .RADIAN. ) );
#9078=CARTESIAN_POINT ( 'NONE',  ( 70.38703763562273252, -92.47916748300480094, 14.88498244535495907 ) ) ;
#9080=CARTESIAN_POINT ( 'NONE',  ( -27.49999999999998934, 0.000000000000000000, 127.7817459305202448 ) ) ;
#9086=VERTEX_POINT ( 'NONE', #19525 ) ;
#9088=FACE_BOUND ( 'NONE', #13458, .T. ) ;
#9095=EDGE_CURVE ( 'NONE', #6917, #295, #16192, .T. ) ;
#9099=DIRECTION ( 'NONE',  ( -6.982962677686266711E-15, 0.000000000000000000, -1.000000000000000000 ) ) ;
#9144=EDGE_CURVE ( 'NONE', #20089, #13453, #16830, .T. ) ;
#9155=CARTESIAN_POINT ( 'NONE',  ( 116.5881606921954017, -25.59923667990641150, 14.88498244535463755 ) ) ;
#9162=VECTOR ( 'NONE', #6212, 1000.000000000000000 ) ;
#9167=ORIENTED_EDGE ( 'NONE', *, *, #3381, .T. ) ;
#9174=CIRCLE ( 'NONE', #12772, 3.224098631618460775 ) ;
#9180=DIRECTION ( 'NONE',  ( 6.982962677686266711E-15, -0.000000000000000000, 1.000000000000000000 ) ) ;
#9188=CARTESIAN_POINT ( 'NONE',  ( -23.23469325536255070, -13.41455640552162443, 39.88498244535561810 ) ) ;
#9199=EDGE_CURVE ( 'NONE', #6070, #1994, #501, .T. ) ;
#9205=AXIS2_PLACEMENT_3D ( 'NONE', #9570, #9668, #1797 ) ;
#9206=DIRECTION ( 'NONE',  ( 6.982962677686266711E-15, 0.000000000000000000, 1.000000000000000000 ) ) ;
#9208=EDGE_LOOP ( 'NONE', ( #16435, #7532, #2009, #10544 ) ) ;
#9210=DIRECTION ( 'NONE',  ( 6.982962677686266711E-15, -0.000000000000000000, 1.000000000000000000 ) ) ;
#9215=DIRECTION ( 'NONE',  ( 1.000000000000000000, 0.000000000000000000, -6.994638739193269649E-15 ) ) ;
#9231=AXIS2_PLACEMENT_3D ( 'NONE', #10743, #5953, #6059 ) ;
#9250=ORIENTED_EDGE ( 'NONE', *, *, #5302, .T. ) ;
#9253=EDGE_CURVE ( 'NONE', #19254, #17576, #1311, .T. ) ;
#9254=CIRCLE ( 'NONE', #15132, 3.224098631618459443 ) ;
#9259=VERTEX_POINT ( 'NONE', #18092 ) ;
#9266=AXIS2_PLACEMENT_3D ( 'NONE', #17300, #9708, #1733 ) ;
#9277=ORIENTED_EDGE ( 'NONE', *, *, #10163, .F. ) ;
#9285=DIRECTION ( 'NONE',  ( 6.982962677686266711E-15, -0.000000000000000000, 1.000000000000000000 ) ) ;
#9287=DIRECTION ( 'NONE',  ( 1.000000000000000000, 0.000000000000000000, -6.994638739193275171E-15 ) ) ;
#9289=ORIENTED_EDGE ( 'NONE', *, *, #11773, .T. ) ;
#9302=DIRECTION ( 'NONE',  ( -6.982962677686266711E-15, 0.000000000000000000, -1.000000000000000000 ) ) ;
#9309=CARTESIAN_POINT ( 'NONE',  ( 12.24586475280392506, -24.22555452564823497, 14.88498244535536585 ) ) ;
#9326=ORIENTED_EDGE ( 'NONE', *, *, #17165, .T. ) ;
#9327=ORIENTED_EDGE ( 'NONE', *, *, #5603, .T. ) ;
#9329=ORIENTED_EDGE ( 'NONE', *, *, #14484, .T. ) ;
#9343=CARTESIAN_POINT ( 'NONE',  ( 19.63382932406824466, 18.38657833536341357, 14.88498244535531256 ) ) ;
#9367=DIRECTION ( 'NONE',  ( -6.982962677686266711E-15, 0.000000000000000000, -1.000000000000000000 ) ) ;
#9377=ORIENTED_EDGE ( 'NONE', *, *, #1371, .F. ) ;
#9456=ORIENTED_EDGE ( 'NONE', *, *, #16313, .F. ) ;
#9469=CYLINDRICAL_SURFACE ( 'NONE', #16623, 3.224098631618460331 ) ;
#9471=CYLINDRICAL_SURFACE ( 'NONE', #1264, 112.8770930172170210 ) ;
#9475=ADVANCED_FACE ( 'NONE', ( #14696 ), #485, .T. ) ;
#9479=ORIENTED_EDGE ( 'NONE', *, *, #8714, .F. ) ;
#9480=ORIENTED_EDGE ( 'NONE', *, *, #17738, .F. ) ;
#9488=DIRECTION ( 'NONE',  ( 0.9396926207859056523, -0.3420201433256757628, -6.584943678403441173E-15 ) ) ;
#9491=DIRECTION ( 'NONE',  ( 0.9396926207859063185, -0.3420201433256742640, -6.456589605409180904E-15 ) ) ;
#9506=CIRCLE ( 'NONE', #14412, 3.224098631618461663 ) ;
#9522=CARTESIAN_POINT ( 'NONE',  ( -5.524863963826822655, -116.0870680293436408, 14.88498244535549020 ) ) ;
#9532=CARTESIAN_POINT ( 'NONE',  ( -97.95177330934026827, 59.60912842347561025, 14.88498244535613502 ) ) ;
#9540=CARTESIAN_POINT ( 'NONE',  ( -1.396592535537253342E-14, 0.000000000000000000, 39.88498244535545467 ) ) ;
#9547=CARTESIAN_POINT ( 'NONE',  ( -17.49999999999999289, 2.143131898507871009E-15, 49.99999999999998579 ) ) ;
#9551=EDGE_CURVE ( 'NONE', #3116, #1080, #8352, .T. ) ;
#9562=VERTEX_POINT ( 'NONE', #13053 ) ;
#9570=CARTESIAN_POINT ( 'NONE',  ( 81.66698895276897474, 79.37254397626031732, 39.88498244535488624 ) ) ;
#9582=ORIENTED_EDGE ( 'NONE', *, *, #16197, .F. ) ;
#9589=CARTESIAN_POINT ( 'NONE',  ( 26.85905058935142975, 1.464553941565464035, 14.88498244535526460 ) ) ;
#9598=DIRECTION ( 'NONE',  ( -0.1736481776669409338, -0.9848077530122062440, 1.076098267568195634E-15 ) ) ;
#9599=CARTESIAN_POINT ( 'NONE',  ( -20.01059462374426445, -13.41455640552162443, 14.88498244535559323 ) ) ;
#9610=EDGE_CURVE ( 'NONE', #8547, #15546, #18944, .T. ) ;
#9619=CYLINDRICAL_SURFACE ( 'NONE', #18323, 106.4288957539801004 ) ;
#9632=EDGE_LOOP ( 'NONE', ( #1331, #4162, #7417, #15373 ) ) ;
#9639=ADVANCED_FACE ( 'NONE', ( #14990 ), #11906, .T. ) ;
#9648=DIRECTION ( 'NONE',  ( 1.000000000000000000, 0.000000000000000000, -6.994638739193275171E-15 ) ) ;
#9650=ORIENTED_EDGE ( 'NONE', *, *, #4242, .T. ) ;
#9655=ORIENTED_EDGE ( 'NONE', *, *, #7511, .F. ) ;
#9668=DIRECTION ( 'NONE',  ( -6.982962677686266711E-15, 0.000000000000000000, -1.000000000000000000 ) ) ;
#9673=ORIENTED_EDGE ( 'NONE', *, *, #13333, .F. ) ;
#9684=CARTESIAN_POINT ( 'NONE',  ( -36.71940246244727035, 108.6254278180370250, 39.88498244535571047 ) ) ;
#9689=CARTESIAN_POINT ( 'NONE',  ( -27.10287801637868199, 1.507547295587424951, 14.88498244535564297 ) ) ;
#9700=ORIENTED_EDGE ( 'NONE', *, *, #16281, .F. ) ;
#9706=DIRECTION ( 'NONE',  ( 6.982962677686266711E-15, 0.000000000000000000, 1.000000000000000000 ) ) ;
#9708=DIRECTION ( 'NONE',  ( 6.982962677686266711E-15, -0.000000000000000000, 1.000000000000000000 ) ) ;
#9732=ORIENTED_EDGE ( 'NONE', *, *, #5285, .T. ) ;
#9735=CARTESIAN_POINT ( 'NONE',  ( 44.89578954330581695, 107.1965464310834477, 14.88498244535514026 ) ) ;
#9740=AXIS2_PLACEMENT_3D ( 'NONE', #691, #6934, #13153 ) ;
#9741=DIRECTION ( 'NONE',  ( 6.982962677686266711E-15, -0.000000000000000000, 1.000000000000000000 ) ) ;
#9742=DIRECTION ( 'NONE',  ( 1.000000000000000000, 0.000000000000000000, -6.994638739193269649E-15 ) ) ;
#9746=FACE_OUTER_BOUND ( 'NONE', #1911, .T. ) ;
#9756=ORIENTED_EDGE ( 'NONE', *, *, #19291, .T. ) ;
#9778=CIRCLE ( 'NONE', #4550, 112.8770930172170068 ) ;
#9800=AXIS2_PLACEMENT_3D ( 'NONE', #3488, #1654, #19052 ) ;
#9814=DIRECTION ( 'NONE',  ( -6.982962677686266711E-15, 0.000000000000000000, -1.000000000000000000 ) ) ;
#9815=LINE ( 'NONE', #2053, #12103 ) ;
#9829=ADVANCED_FACE ( 'NONE', ( #12524 ), #20099, .F. ) ;
#9831=VERTEX_POINT ( 'NONE', #9155 ) ;
#9842=DIRECTION ( 'NONE',  ( -0.7660444431189857850, -0.6427876096865300370, 5.348151281215662765E-15 ) ) ;
#9846=DIRECTION ( 'NONE',  ( 1.000000000000000000, 0.000000000000000000, -0.000000000000000000 ) ) ;
#9865=FACE_OUTER_BOUND ( 'NONE', #2636, .T. ) ;
#9869=CARTESIAN_POINT ( 'NONE',  ( 100.5989061668482520, 55.02415981988612970, 14.88498244535475123 ) ) ;
#9873=EDGE_CURVE ( 'NONE', #16155, #15471, #15336, .T. ) ;
#9881=ORIENTED_EDGE ( 'NONE', *, *, #17752, .T. ) ;
#9885=CARTESIAN_POINT ( 'NONE',  ( -1.396592535537253342E-14, 0.000000000000000000, 39.88498244535545467 ) ) ;
#9907=ORIENTED_EDGE ( 'NONE', *, *, #2589, .T. ) ;
#9923=DIRECTION ( 'NONE',  ( 6.982962677686266711E-15, -0.000000000000000000, 1.000000000000000000 ) ) ;
#9925=PLANE ( 'NONE',  #11531 ) ;
#9932=CARTESIAN_POINT ( 'NONE',  ( -63.98537287693041264, 94.20918150411493741, 14.88498244535589876 ) ) ;
#9951=AXIS2_PLACEMENT_3D ( 'NONE', #6155, #15559, #15452 ) ;
#9955=ORIENTED_EDGE ( 'NONE', *, *, #4320, .T. ) ;
#9962=AXIS2_PLACEMENT_3D ( 'NONE', #13633, #7106, #10562 ) ;
#9990=CARTESIAN_POINT ( 'NONE',  ( 1.396592535537253342E-14, 0.000000000000000000, 43.88498244535545467 ) ) ;
#9995=DIRECTION ( 'NONE',  ( -1.000000000000000000, 0.000000000000000000, 6.976128451377903642E-15 ) ) ;
#10023=CARTESIAN_POINT ( 'NONE',  ( 105.9946577255053626, 51.49356311920430329, 14.88498244535471215 ) ) ;
#10025=DIRECTION ( 'NONE',  ( 6.982962677686266711E-15, -0.000000000000000000, 1.000000000000000000 ) ) ;
#10052=AXIS2_PLACEMENT_3D ( 'NONE', #4281, #16762, #12249 ) ;
#10072=CIRCLE ( 'NONE', #8161, 112.8770930172170495 ) ;
#10093=CARTESIAN_POINT ( 'NONE',  ( -26.42151830275515323, 4.658826548058537576, 14.88498244535563586 ) ) ;
#10096=EDGE_CURVE ( 'NONE', #9086, #16353, #13369, .T. ) ;
#10115=CYLINDRICAL_SURFACE ( 'NONE', #18484, 112.8770930172170210 ) ;
#10116=DIRECTION ( 'NONE',  ( -0.7660444431189772363, 0.6427876096865402511, 4.304393070272779381E-15 ) ) ;
#10132=PLANE ( 'NONE',  #10722 ) ;
#10135=ORIENTED_EDGE ( 'NONE', *, *, #8577, .F. ) ;
#10145=VECTOR ( 'NONE', #3638, 1000.000000000000000 ) ;
#10150=DIRECTION ( 'NONE',  ( -1.000000000000000000, 0.000000000000000000, 6.977185866873309606E-15 ) ) ;
#10156=EDGE_CURVE ( 'NONE', #6223, #19500, #2493, .T. ) ;
#10163=EDGE_CURVE ( 'NONE', #19981, #7250, #18625, .T. ) ;
#10211=CIRCLE ( 'NONE', #14468, 3.224098631618460331 ) ;
#10215=ORIENTED_EDGE ( 'NONE', *, *, #19993, .F. ) ;
#10221=CARTESIAN_POINT ( 'NONE',  ( -34.51244174799990816, 110.9757759606085017, 14.88498244535569093 ) ) ;
#10225=EDGE_CURVE ( 'NONE', #14181, #1862, #3598, .T. ) ;
#10232=EDGE_LOOP ( 'NONE', ( #49, #8814, #15825, #17795 ) ) ;
#10233=AXIS2_PLACEMENT_3D ( 'NONE', #17038, #5072, #456 ) ;
#10238=DIRECTION ( 'NONE',  ( -0.1736481776669404620, -0.9848077530122062440, 1.212578743696479242E-15 ) ) ;
#10261=DIRECTION ( 'NONE',  ( -6.982962677686266711E-15, 0.000000000000000000, -1.000000000000000000 ) ) ;
#10273=ADVANCED_FACE ( 'NONE', ( #15372 ), #1361, .T. ) ;
#10276=CARTESIAN_POINT ( 'NONE',  ( 70.38703763562291726, -92.47916748300480094, 39.88498244535495729 ) ) ;
#10278=CARTESIAN_POINT ( 'NONE',  ( -127.4413876050234933, 1.560706874093891490E-14, 39.88498244535634285 ) ) ;
#10291=CYLINDRICAL_SURFACE ( 'NONE', #10985, 3.224098631618460331 ) ;
#10292=ORIENTED_EDGE ( 'NONE', *, *, #7366, .F. ) ;
#10300=CARTESIAN_POINT ( 'NONE',  ( -21.73104181959847025, -16.26654594725001957, 14.88498244535560389 ) ) ;
#10303=CIRCLE ( 'NONE', #4429, 112.8770930172170495 ) ;
#10329=PLANE ( 'NONE',  #10569 ) ;
#10333=DIRECTION ( 'NONE',  ( -0.000000000000000000, -0.000000000000000000, -1.000000000000000000 ) ) ;
#10348=VECTOR ( 'NONE', #18716, 1000.000000000000000 ) ;
#10351=CARTESIAN_POINT ( 'NONE',  ( 113.5802308907675666, 8.308367629983374414, 14.88498244535465709 ) ) ;
#10366=ORIENTED_EDGE ( 'NONE', *, *, #14168, .F. ) ;
#10375=ORIENTED_EDGE ( 'NONE', *, *, #15664, .T. ) ;
#10377=FACE_OUTER_BOUND ( 'NONE', #5333, .T. ) ;
#10385=EDGE_LOOP ( 'NONE', ( #20143, #19083, #15925, #9756 ) ) ;
#10407=AXIS2_PLACEMENT_3D ( 'NONE', #1067, #16636, #1170 ) ;
#10413=CYLINDRICAL_SURFACE ( 'NONE', #1727, 106.4288957539801004 ) ;
#10416=FACE_BOUND ( 'NONE', #13242, .T. ) ;
#10424=DIRECTION ( 'NONE',  ( 6.982962677686266711E-15, -0.000000000000000000, 1.000000000000000000 ) ) ;
#10431=CARTESIAN_POINT ( 'NONE',  ( 103.2967819461768073, 53.25886146954521649, 14.88498244535472992 ) ) ;
#10450=VERTEX_POINT ( 'NONE', #11831 ) ;
#10451=DIRECTION ( 'NONE',  ( -6.982962677686266711E-15, 0.000000000000000000, -1.000000000000000000 ) ) ;
#10453=CARTESIAN_POINT ( 'NONE',  ( 69.11703934647968595, -95.44259730872654757, 39.88498244535497150 ) ) ;
#10460=LINE ( 'NONE', #3757, #4660 ) ;
#10461=VECTOR ( 'NONE', #19721, 1000.000000000000000 ) ;
#10500=ORIENTED_EDGE ( 'NONE', *, *, #17420, .F. ) ;
#10530=CARTESIAN_POINT ( 'NONE',  ( 103.2967819461768073, 53.25886146954521649, 14.88498244535472992 ) ) ;
#10531=CARTESIAN_POINT ( 'NONE',  ( -3.143238168843667690, 31.03941509555038181, 14.88498244535547599 ) ) ;
#10544=ORIENTED_EDGE ( 'NONE', *, *, #3964, .F. ) ;
#10550=CYLINDRICAL_SURFACE ( 'NONE', #7422, 106.4288957539801004 ) ;
#10552=AXIS2_PLACEMENT_3D ( 'NONE', #4387, #19934, #7354 ) ;
#10559=CIRCLE ( 'NONE', #18083, 3.224098631618459443 ) ;
#10562=DIRECTION ( 'NONE',  ( -0.1736481776669404065, -0.9848077530122062440, 1.238751781085795583E-15 ) ) ;
#10568=ORIENTED_EDGE ( 'NONE', *, *, #15664, .F. ) ;
#10569=AXIS2_PLACEMENT_3D ( 'NONE', #14751, #734, #10238 ) ;
#10570=ADVANCED_FACE ( 'NONE', ( #12247 ), #4378, .T. ) ;
#10579=CARTESIAN_POINT ( 'NONE',  ( 12.24586475280413289, -24.22555452564822787, 39.88498244535536941 ) ) ;
#10620=ORIENTED_EDGE ( 'NONE', *, *, #14791, .F. ) ;
#10623=DIRECTION ( 'NONE',  ( 6.982962677686266711E-15, -0.000000000000000000, 1.000000000000000000 ) ) ;
#10651=ORIENTED_EDGE ( 'NONE', *, *, #1543, .T. ) ;
#10657=DIRECTION ( 'NONE',  ( 0.9396926207859104263, 0.3420201433256629953, -6.568644312862836368E-15 ) ) ;
#10660=CARTESIAN_POINT ( 'NONE',  ( -5.524863963826648572, -116.0870680293436408, 39.88498244535549730 ) ) ;
#10662=CIRCLE ( 'NONE', #16551, 112.8770930172170495 ) ;
#10676=CARTESIAN_POINT ( 'NONE',  ( -12.16118437606778535, -23.99289710269258080, 14.88498244535553461 ) ) ;
#10722=AXIS2_PLACEMENT_3D ( 'NONE', #6961, #11940, #13181 ) ;
#10728=VERTEX_POINT ( 'NONE', #6439 ) ;
#10740=ORIENTED_EDGE ( 'NONE', *, *, #16251, .T. ) ;
#10743=CARTESIAN_POINT ( 'NONE',  ( 1.378965026025638009E-14, 26.82911281104372847, 39.88498244535545467 ) ) ;
#10762=ADVANCED_FACE ( 'NONE', ( #19217 ), #15943, .T. ) ;
#10779=CIRCLE ( 'NONE', #979, 3.224098631618460331 ) ;
#10780=VERTEX_POINT ( 'NONE', #19317 ) ;
#10783=PLANE ( 'NONE',  #10233 ) ;
#10829=ORIENTED_EDGE ( 'NONE', *, *, #18017, .T. ) ;
#10835=EDGE_CURVE ( 'NONE', #16647, #16902, #16629, .T. ) ;
#10837=EDGE_LOOP ( 'NONE', ( #8295, #10215 ) ) ;
#10838=DIRECTION ( 'NONE',  ( 6.982962677686266711E-15, -0.000000000000000000, 1.000000000000000000 ) ) ;
#10892=CARTESIAN_POINT ( 'NONE',  ( -1.396592535537253342E-14, 0.000000000000000000, 39.88498244535545467 ) ) ;
#10905=VERTEX_POINT ( 'NONE', #4252 ) ;
#10906=DIRECTION ( 'NONE',  ( -0.1736481776669273613, 0.9848077530122086864, 1.212578743696387931E-15 ) ) ;
#10913=CARTESIAN_POINT ( 'NONE',  ( -5.524863963826648572, -116.0870680293436408, 39.88498244535549730 ) ) ;
#10922=DIRECTION ( 'NONE',  ( -0.000000000000000000, -0.000000000000000000, -1.000000000000000000 ) ) ;
#10924=DIRECTION ( 'NONE',  ( 0.4999999999999916178, -0.8660254037844435926, -4.304393070272782536E-15 ) ) ;
#10937=VERTEX_POINT ( 'NONE', #10579 ) ;
#10945=CIRCLE ( 'NONE', #504, 106.4288957539801146 ) ;
#10957=VERTEX_POINT ( 'NONE', #15193 ) ;
#10963=DIRECTION ( 'NONE',  ( -1.000000000000000000, 0.000000000000000000, 6.977185866873309606E-15 ) ) ;
#10985=AXIS2_PLACEMENT_3D ( 'NONE', #6936, #19422, #5403 ) ;
#10991=DIRECTION ( 'NONE',  ( 6.982962677686266711E-15, -0.000000000000000000, 1.000000000000000000 ) ) ;
#10995=AXIS2_PLACEMENT_3D ( 'NONE', #11807, #7129, #16342 ) ;
#11000=ORIENTED_EDGE ( 'NONE', *, *, #13031, .F. ) ;
#11019=ADVANCED_FACE ( 'NONE', ( #2930 ), #9471, .T. ) ;
#11020=AXIS2_PLACEMENT_3D ( 'NONE', #13059, #12960, #11627 ) ;
#11044=ADVANCED_FACE ( 'NONE', ( #14070 ), #20207, .T. ) ;
#11051=CARTESIAN_POINT ( 'NONE',  ( 127.4413876050234364, 0.000000000000000000, 39.88498244535456649 ) ) ;
#11057=EDGE_LOOP ( 'NONE', ( #11468, #5470, #17465, #11117, #5604 ) ) ;
#11062=ORIENTED_EDGE ( 'NONE', *, *, #18300, .F. ) ;
#11076=DIRECTION ( 'NONE',  ( 0.000000000000000000, 0.000000000000000000, 1.000000000000000000 ) ) ;
#11092=ORIENTED_EDGE ( 'NONE', *, *, #5603, .F. ) ;
#11097=LINE ( 'NONE', #9869, #11676 ) ;
#11101=FACE_OUTER_BOUND ( 'NONE', #19224, .T. ) ;
#11116=DIRECTION ( 'NONE',  ( 6.982962677686266711E-15, -0.000000000000000000, 1.000000000000000000 ) ) ;
#11117=ORIENTED_EDGE ( 'NONE', *, *, #4376, .T. ) ;
#11141=DIRECTION ( 'NONE',  ( -6.982962677686266711E-15, 0.000000000000000000, -1.000000000000000000 ) ) ;
#11169=CIRCLE ( 'NONE', #8566, 106.4288957539801430 ) ;
#11182=CIRCLE ( 'NONE', #18365, 3.224098631618460331 ) ;
#11185=CIRCLE ( 'NONE', #2372, 106.4288957539801004 ) ;
#11190=DIRECTION ( 'NONE',  ( -0.7660444431189770143, 0.6427876096865404731, 5.346191897317644801E-15 ) ) ;
#11209=EDGE_CURVE ( 'NONE', #17841, #19703, #16020, .T. ) ;
#11240=CARTESIAN_POINT ( 'NONE',  ( -49.59485801383857506, -102.5175491340983882, 14.88498244535579929 ) ) ;
#11245=CARTESIAN_POINT ( 'NONE',  ( 17.50000000000001776, 0.000000000000000000, 49.99999999999998579 ) ) ;
#11248=DIRECTION ( 'NONE',  ( 6.982962677686266711E-15, -0.000000000000000000, 1.000000000000000000 ) ) ;
#11267=VERTEX_POINT ( 'NONE', #17327 ) ;
#11282=DIRECTION ( 'NONE',  ( 6.982962677686266711E-15, -0.000000000000000000, 1.000000000000000000 ) ) ;
#11291=EDGE_CURVE ( 'NONE', #6744, #13679, #4908, .T. ) ;
#11297=DIRECTION ( 'NONE',  ( 6.982962677686266711E-15, 0.000000000000000000, 1.000000000000000000 ) ) ;
#11303=FACE_OUTER_BOUND ( 'NONE', #3899, .T. ) ;
#11304=DIRECTION ( 'NONE',  ( -0.7660444431189858960, -0.6427876096865298150, 5.346191897317643224E-15 ) ) ;
#11319=AXIS2_PLACEMENT_3D ( 'NONE', #2432, #14899, #5497 ) ;
#11320=EDGE_LOOP ( 'NONE', ( #12844, #9326, #11497, #17901 ) ) ;
#11337=LINE ( 'NONE', #1630, #10348 ) ;
#11359=DIRECTION ( 'NONE',  ( -0.7660444431189865622, -0.6427876096865291489, 5.380491337840971071E-15 ) ) ;
#11372=EDGE_CURVE ( 'NONE', #15086, #141, #3908, .T. ) ;
#11375=DIRECTION ( 'NONE',  ( -6.982962677686266711E-15, 0.000000000000000000, -1.000000000000000000 ) ) ;
#11377=ORIENTED_EDGE ( 'NONE', *, *, #15761, .T. ) ;
#11387=CARTESIAN_POINT ( 'NONE',  ( 44.89578954330581695, 107.1965464310834477, 14.88498244535514026 ) ) ;
#11392=AXIS2_PLACEMENT_3D ( 'NONE', #9078, #15321, #1200 ) ;
#11420=AXIS2_PLACEMENT_3D ( 'NONE', #15779, #4842, #14036 ) ;
#11435=DIRECTION ( 'NONE',  ( -0.7660444431189862291, -0.6427876096865298150, 4.304393070272780959E-15 ) ) ;
#11440=ORIENTED_EDGE ( 'NONE', *, *, #9095, .F. ) ;
#11456=DIRECTION ( 'NONE',  ( 0.9396926207859063185, -0.3420201433256742640, -6.456589605409180904E-15 ) ) ;
#11461=CARTESIAN_POINT ( 'NONE',  ( -109.5721339228235820, 31.03941509555038181, 39.88498244535622206 ) ) ;
#11467=ORIENTED_EDGE ( 'NONE', *, *, #3272, .F. ) ;
#11468=ORIENTED_EDGE ( 'NONE', *, *, #16774, .T. ) ;
#11478=CARTESIAN_POINT ( 'NONE',  ( 114.2960429025578293, -28.68569479505797659, 39.88498244535465176 ) ) ;
#11482=SHAPE_REPRESENTATION_RELATIONSHIP ( 'NONE' , 'NONE' ,  #5472, #15283 ) ;
#11483=FACE_BOUND ( 'NONE', #15137, .T. ) ;
#11495=DIRECTION ( 'NONE',  ( -0.7660444431189865622, -0.6427876096865291489, 4.304393070272777014E-15 ) ) ;
#11497=ORIENTED_EDGE ( 'NONE', *, *, #16188, .T. ) ;
#11507=EDGE_CURVE ( 'NONE', #18211, #9562, #10072, .T. ) ;
#11508=VERTEX_POINT ( 'NONE', #2562 ) ;
#11509=ORIENTED_EDGE ( 'NONE', *, *, #13991, .F. ) ;
#11514=EDGE_CURVE ( 'NONE', #912, #2184, #18113, .T. ) ;
#11527=DIRECTION ( 'NONE',  ( 6.982962677686266711E-15, -0.000000000000000000, 1.000000000000000000 ) ) ;
#11530=ADVANCED_FACE ( 'NONE', ( #7263 ), #13487, .T. ) ;
#11531=AXIS2_PLACEMENT_3D ( 'NONE', #2262, #19532, #17614 ) ;
#11533=DIRECTION ( 'NONE',  ( -6.982962677686266711E-15, 0.000000000000000000, -1.000000000000000000 ) ) ;
#11550=ORIENTED_EDGE ( 'NONE', *, *, #5881, .T. ) ;
#11553=AXIS2_PLACEMENT_3D ( 'NONE', #5267, #17744, #5363 ) ;
#11565=ORIENTED_EDGE ( 'NONE', *, *, #7018, .T. ) ;
#11589=ORIENTED_EDGE ( 'NONE', *, *, #15239, .F. ) ;
#11599=DIRECTION ( 'NONE',  ( 0.9396926207859105373, 0.3420201433256631063, -6.577611345862942596E-15 ) ) ;
#11627=DIRECTION ( 'NONE',  ( 0.9396926207859058744, -0.3420201433256756518, -6.577611345862941807E-15 ) ) ;
#11640=CLOSED_SHELL ( 'NONE', ( #3237, #105, #10273, #15293, #17789, #3046, #17131, #16303, #17007, #4747, #2834, #12112, #12404, #7668, #11044, #19629, #18219, #3482, #6511, #4653, #17887, #17667, #6683, #16501, #8093, #19416, #7795, #3423, #14024, #7335, #6870, #15790, #16053, #13707, #5506, #5981, #7132, #7284, #18145, #10570, #851, #3802, #9829, #10762, #8494, #11019, #11530, #14101, #7628, #16922, #8345, #19787, #6052, #7264, #16990, #9639, #9475, #15091, #14721, #14174, #12138, #18564, #19284, #15995, #5717, #2987 ) ) ;
#11652=DIRECTION ( 'NONE',  ( 6.982962677686266711E-15, -0.000000000000000000, 1.000000000000000000 ) ) ;
#11655=AXIS2_PLACEMENT_3D ( 'NONE', #2929, #2722, #4562 ) ;
#11658=FACE_OUTER_BOUND ( 'NONE', #4177, .T. ) ;
#11661=AXIS2_PLACEMENT_3D ( 'NONE', #14826, #11652, #2163 ) ;
#11673=CARTESIAN_POINT ( 'NONE',  ( -32.30548103355219780, 113.3261241031799926, 39.88498244535568205 ) ) ;
#11676=VECTOR ( 'NONE', #1801, 1000.000000000000000 ) ;
#11684=VECTOR ( 'NONE', #362, 1000.000000000000000 ) ;
#11714=CYLINDRICAL_SURFACE ( 'NONE', #10995, 17.50000000000000355 ) ;
#11730=ORIENTED_EDGE ( 'NONE', *, *, #11873, .T. ) ;
#11748=VERTEX_POINT ( 'NONE', #3474 ) ;
#11752=CIRCLE ( 'NONE', #16996, 3.224098631618459443 ) ;
#11768=CARTESIAN_POINT ( 'NONE',  ( 41.69438488732666315, 106.8146822993833780, 14.88498244535515980 ) ) ;
#11773=EDGE_CURVE ( 'NONE', #3116, #2014, #7185, .T. ) ;
#11784=CARTESIAN_POINT ( 'NONE',  ( 23.23469325536231622, -13.41455640552199924, 39.88498244535529125 ) ) ;
#11786=CARTESIAN_POINT ( 'NONE',  ( -27.49999999999998934, 0.000000000000000000, 43.88498244535566073 ) ) ;
#11795=ORIENTED_EDGE ( 'NONE', *, *, #14653, .T. ) ;
#11807=CARTESIAN_POINT ( 'NONE',  ( -1.396592535537253342E-14, 0.000000000000000000, 39.88498244535545467 ) ) ;
#11813=EDGE_CURVE ( 'NONE', #1994, #6070, #3863, .T. ) ;
#11815=AXIS2_PLACEMENT_3D ( 'NONE', #8561, #11533, #16253 ) ;
#11827=DIRECTION ( 'NONE',  ( 6.982962677686266711E-15, -0.000000000000000000, 1.000000000000000000 ) ) ;
#11829=VERTEX_POINT ( 'NONE', #11922 ) ;
#11831=CARTESIAN_POINT ( 'NONE',  ( 3.304959094393419949, 31.03941509555038181, 39.88498244535543336 ) ) ;
#11840=DIRECTION ( 'NONE',  ( -0.1736481776669280275, 0.9848077530122084644, 1.076098267568195831E-15 ) ) ;
#11860=DIRECTION ( 'NONE',  ( -1.000000000000000000, 0.000000000000000000, 0.000000000000000000 ) ) ;
#11861=CARTESIAN_POINT ( 'NONE',  ( -103.8888757476053541, -46.65403860089418941, 14.88498244535617765 ) ) ;
#11864=CARTESIAN_POINT ( 'NONE',  ( -1.607844166819003129E-13, 26.82911281104372847, 14.88498244535545112 ) ) ;
#11873=EDGE_CURVE ( 'NONE', #2341, #8253, #994, .T. ) ;
#11874=EDGE_CURVE ( 'NONE', #4820, #16400, #3548, .T. ) ;
#11882=AXIS2_PLACEMENT_3D ( 'NONE', #9522, #3286, #11456 ) ;
#11891=ORIENTED_EDGE ( 'NONE', *, *, #5156, .F. ) ;
#11893=AXIS2_PLACEMENT_3D ( 'NONE', #16855, #9180, #9287 ) ;
#11897=ORIENTED_EDGE ( 'NONE', *, *, #9095, .T. ) ;
#11898=EDGE_LOOP ( 'NONE', ( #12674, #17483, #11992, #6893 ) ) ;
#11906=CYLINDRICAL_SURFACE ( 'NONE', #10407, 112.8770930172170210 ) ;
#11916=ORIENTED_EDGE ( 'NONE', *, *, #17334, .T. ) ;
#11918=ORIENTED_EDGE ( 'NONE', *, *, #19716, .T. ) ;
#11920=ORIENTED_EDGE ( 'NONE', *, *, #15775, .T. ) ;
#11922=CARTESIAN_POINT ( 'NONE',  ( 21.51662357878014831, -16.14275151819498078, 39.88498244535530546 ) ) ;
#11923=SURFACE_SIDE_STYLE ('',( #17064 ) ) ;
#11928=ORIENTED_EDGE ( 'NONE', *, *, #5881, .F. ) ;
#11940=DIRECTION ( 'NONE',  ( -6.982962677686267499E-15, -3.944304526105059027E-31, -1.000000000000000000 ) ) ;
#11943=AXIS2_PLACEMENT_3D ( 'NONE', #18266, #12313, #1066 ) ;
#11947=ORIENTED_EDGE ( 'NONE', *, *, #11813, .F. ) ;
#11948=CARTESIAN_POINT ( 'NONE',  ( -9.176097008934114285, -25.21111933077039069, 14.88498244535551507 ) ) ;
#11959=CARTESIAN_POINT ( 'NONE',  ( 70.38703763562273252, -92.47916748300480094, 14.88498244535495907 ) ) ;
#11975=ORIENTED_EDGE ( 'NONE', *, *, #5156, .T. ) ;
#11978=CARTESIAN_POINT ( 'NONE',  ( -97.59206265536077751, 66.04728469612305730, 14.88498244535613146 ) ) ;
#11992=ORIENTED_EDGE ( 'NONE', *, *, #17752, .F. ) ;
#11998=AXIS2_PLACEMENT_3D ( 'NONE', #16896, #4412, #9215 ) ;
#12021=DIRECTION ( 'NONE',  ( -6.982962677686266711E-15, 0.000000000000000000, -1.000000000000000000 ) ) ;
#12025=EDGE_CURVE ( 'NONE', #3088, #7939, #1261, .T. ) ;
#12027=CARTESIAN_POINT ( 'NONE',  ( -17.50000000000001776, 2.143131898507872981E-15, 39.88498244535557546 ) ) ;
#12034=ORIENTED_EDGE ( 'NONE', *, *, #8577, .T. ) ;
#12065=FACE_OUTER_BOUND ( 'NONE', #10232, .T. ) ;
#12071=ORIENTED_EDGE ( 'NONE', *, *, #16107, .T. ) ;
#12075=PRODUCT_DEFINITION_FORMATION_WITH_SPECIFIED_SOURCE ( 'ANY', '', #3622, .NOT_KNOWN. ) ;
#12101=EDGE_LOOP ( 'NONE', ( #9377, #3099, #9907, #5891 ) ) ;
#12103=VECTOR ( 'NONE', #19136, 1000.000000000000000 ) ;
#12112=ADVANCED_FACE ( 'NONE', ( #16605 ), #10550, .F. ) ;
#12114=CARTESIAN_POINT ( 'NONE',  ( 116.5881606921955864, -25.59923667990641150, 39.88498244535464465 ) ) ;
#12117=CARTESIAN_POINT ( 'NONE',  ( 69.11703934647950121, -95.44259730872654757, 14.88498244535496973 ) ) ;
#12128=VERTEX_POINT ( 'NONE', #1461 ) ;
#12131=CARTESIAN_POINT ( 'NONE',  ( -27.10287801637851501, 1.507547295587399638, 39.88498244535563941 ) ) ;
#12138=ADVANCED_FACE ( 'NONE', ( #19918 ), #4472, .T. ) ;
#12144=CIRCLE ( 'NONE', #11815, 112.8770930172170210 ) ;
#12145=VECTOR ( 'NONE', #12932, 1000.000000000000000 ) ;
#12150=DIRECTION ( 'NONE',  ( -6.982962677686266711E-15, 0.000000000000000000, -1.000000000000000000 ) ) ;
#12161=ORIENTED_EDGE ( 'NONE', *, *, #15502, .T. ) ;
#12162=AXIS2_PLACEMENT_3D ( 'NONE', #8806, #6056, #9002 ) ;
#12190=AXIS2_PLACEMENT_3D ( 'NONE', #9932, #15031, #16181 ) ;
#12199=DIRECTION ( 'NONE',  ( -6.982962677686266711E-15, 0.000000000000000000, -1.000000000000000000 ) ) ;
#12204=COLOUR_RGB ( '', 0.31764706, 0.68627451, 0.89019608) ;
#12218=EDGE_CURVE ( 'NONE', #9259, #1807, #12990, .T. ) ;
#12232=EDGE_LOOP ( 'NONE', ( #5339, #5558, #9167, #18151 ) ) ;
#12247=FACE_OUTER_BOUND ( 'NONE', #18697, .T. ) ;
#12249=DIRECTION ( 'NONE',  ( 1.000000000000000000, 0.000000000000000000, -6.994638739193269649E-15 ) ) ;
#12251=AXIS2_PLACEMENT_3D ( 'NONE', #4928, #19134, #17505 ) ;
#12274=DIRECTION ( 'NONE',  ( 6.982962677686266711E-15, -0.000000000000000000, 1.000000000000000000 ) ) ;
#12278=AXIS2_PLACEMENT_3D ( 'NONE', #6288, #8380, #3312 ) ;
#12313=DIRECTION ( 'NONE',  ( -0.000000000000000000, -0.000000000000000000, -1.000000000000000000 ) ) ;
#12317=DIRECTION ( 'NONE',  ( 1.000000000000000000, 0.000000000000000000, -6.976128451377902853E-15 ) ) ;
#12325=CARTESIAN_POINT ( 'NONE',  ( -5.951998377315478983, -25.21111933077039069, 39.88498244535549730 ) ) ;
#12331=DIRECTION ( 'NONE',  ( -6.982962677686266711E-15, 1.972152263052529076E-31, -1.000000000000000000 ) ) ;
#12339=ORIENTED_EDGE ( 'NONE', *, *, #2499, .T. ) ;
#12348=EDGE_CURVE ( 'NONE', #7939, #14390, #2538, .T. ) ;
#12359=PLANE ( 'NONE',  #16600 ) ;
#12365=ORIENTED_EDGE ( 'NONE', *, *, #13031, .T. ) ;
#12370=CARTESIAN_POINT ( 'NONE',  ( -8.402595070145098433, -117.5408478153264298, 14.88498244535551152 ) ) ;
#12379=FACE_OUTER_BOUND ( 'NONE', #2138, .T. ) ;
#12384=CYLINDRICAL_SURFACE ( 'NONE', #11998, 3.224098631618460331 ) ;
#12404=ADVANCED_FACE ( 'NONE', ( #19015 ), #3153, .T. ) ;
#12408=DIRECTION ( 'NONE',  ( -1.000000000000000000, 0.000000000000000000, 7.137148015447434001E-15 ) ) ;
#12427=DIRECTION ( 'NONE',  ( 6.982962677686266711E-15, -0.000000000000000000, 1.000000000000000000 ) ) ;
#12442=VECTOR ( 'NONE', #7809, 1000.000000000000000 ) ;
#12449=ORIENTED_EDGE ( 'NONE', *, *, #10163, .T. ) ;
#12462=EDGE_CURVE ( 'NONE', #141, #12565, #6329, .T. ) ;
#12484=ORIENTED_EDGE ( 'NONE', *, *, #4894, .F. ) ;
#12485=EDGE_CURVE ( 'NONE', #12798, #6114, #891, .T. ) ;
#12512=ORIENTED_EDGE ( 'NONE', *, *, #16281, .T. ) ;
#12524=FACE_OUTER_BOUND ( 'NONE', #3669, .T. ) ;
#12527=CARTESIAN_POINT ( 'NONE',  ( 71.65703592476599226, -89.51573765728305432, 14.88498244535495196 ) ) ;
#12547=CARTESIAN_POINT ( 'NONE',  ( 92.34802049131702972, -66.64338626758360817, 39.88498244535480808 ) ) ;
#12557=FACE_OUTER_BOUND ( 'NONE', #11320, .T. ) ;
#12564=CIRCLE ( 'NONE', #19789, 3.224098631618461219 ) ;
#12565=VERTEX_POINT ( 'NONE', #5294 ) ;
#12594=EDGE_CURVE ( 'NONE', #3496, #6273, #16298, .T. ) ;
#12648=FACE_OUTER_BOUND ( 'NONE', #1427, .T. ) ;
#12651=DIRECTION ( 'NONE',  ( 6.982962677686266711E-15, -0.000000000000000000, 1.000000000000000000 ) ) ;
#12674=ORIENTED_EDGE ( 'NONE', *, *, #3272, .T. ) ;
#12691=CARTESIAN_POINT ( 'NONE',  ( 42.44352287704968063, 94.20918150411493741, 14.88498244535515624 ) ) ;
#12707=FACE_OUTER_BOUND ( 'NONE', #10385, .T. ) ;
#12713=DIRECTION ( 'NONE',  ( 0.5000000000000039968, 0.8660254037844362651, -3.228294802704583747E-15 ) ) ;
#12714=AXIS2_PLACEMENT_3D ( 'NONE', #8500, #11375, #17630 ) ;
#12731=EDGE_LOOP ( 'NONE', ( #2261, #3319, #14213, #18596 ) ) ;
#12757=CIRCLE ( 'NONE', #47, 3.224098631618459443 ) ;
#12772=AXIS2_PLACEMENT_3D ( 'NONE', #759, #2308, #16520 ) ;
#12790=DIRECTION ( 'NONE',  ( 6.982962677686266711E-15, -0.000000000000000000, 1.000000000000000000 ) ) ;
#12798=VERTEX_POINT ( 'NONE', #6404 ) ;
#12806=AXIS2_PLACEMENT_3D ( 'NONE', #4770, #3729, #13121 ) ;
#12821=VECTOR ( 'NONE', #4101, 1000.000000000000000 ) ;
#12827=VECTOR ( 'NONE', #8522, 1000.000000000000000 ) ;
#12844=ORIENTED_EDGE ( 'NONE', *, *, #520, .F. ) ;
#12869=ORIENTED_EDGE ( 'NONE', *, *, #4364, .T. ) ;
#12899=ORIENTED_EDGE ( 'NONE', *, *, #14168, .T. ) ;
#12904=ORIENTED_EDGE ( 'NONE', *, *, #16801, .T. ) ;
#12907=CARTESIAN_POINT ( 'NONE',  ( -78.85162031257831927, -85.37653928070189124, 39.88498244535600890 ) ) ;
#12910=CARTESIAN_POINT ( 'NONE',  ( 24.95276293194433492, -10.68636129284900704, 14.88498244535527881 ) ) ;
#12923=VERTEX_POINT ( 'NONE', #13313 ) ;
#12932=DIRECTION ( 'NONE',  ( 6.982962677686266711E-15, -0.000000000000000000, 1.000000000000000000 ) ) ;
#12957=CARTESIAN_POINT ( 'NONE',  ( -109.5721339228237667, 31.03941509555038181, 14.88498244535621851 ) ) ;
#12960=DIRECTION ( 'NONE',  ( -6.982962677686266711E-15, 0.000000000000000000, -1.000000000000000000 ) ) ;
#12963=ORIENTED_EDGE ( 'NONE', *, *, #896, .F. ) ;
#12971=DIRECTION ( 'NONE',  ( -0.1736481776669404897, -0.9848077530122062440, 1.206153050004590509E-15 ) ) ;
#12990=CIRCLE ( 'NONE', #14936, 112.8770930172170068 ) ;
#13003=EDGE_CURVE ( 'NONE', #18698, #7038, #8115, .T. ) ;
#13031=EDGE_CURVE ( 'NONE', #7290, #10780, #1918, .T. ) ;
#13048=DIRECTION ( 'NONE',  ( 1.000000000000000000, 0.000000000000000000, 0.000000000000000000 ) ) ;
#13053=CARTESIAN_POINT ( 'NONE',  ( 21.51662357877997422, -16.14275151819498078, 14.88498244535530191 ) ) ;
#13059=CARTESIAN_POINT ( 'NONE',  ( 92.34802049131702972, -66.64338626758360817, 39.88498244535480808 ) ) ;
#13072=CARTESIAN_POINT ( 'NONE',  ( 48.89172014028660129, 94.20918150411493741, 14.88498244535511184 ) ) ;
#13076=DIRECTION ( 'NONE',  ( 6.982962677686266711E-15, -0.000000000000000000, 1.000000000000000000 ) ) ;
#13084=VECTOR ( 'NONE', #18691, 1000.000000000000000 ) ;
#13089=DIRECTION ( 'NONE',  ( 1.000000000000000000, 0.000000000000000000, -6.994638739193269649E-15 ) ) ;
#13102=CARTESIAN_POINT ( 'NONE',  ( -24.73834469112697576, -10.56256686379325593, 14.88498244535562520 ) ) ;
#13106=DIRECTION ( 'NONE',  ( 6.982962677686266711E-15, 0.000000000000000000, 1.000000000000000000 ) ) ;
#13116=CARTESIAN_POINT ( 'NONE',  ( -97.77191798235034526, 62.82820655979934088, 39.88498244535613679 ) ) ;
#13121=DIRECTION ( 'NONE',  ( 1.000000000000000000, 0.000000000000000000, -6.977185866873308817E-15 ) ) ;
#13124=PRODUCT_DEFINITION_CONTEXT ( 'detailed design', #17313, 'design' ) ;
#13131=ORIENTED_EDGE ( 'NONE', *, *, #478, .T. ) ;
#13141=DIRECTION ( 'NONE',  ( -6.982962677686266711E-15, 0.000000000000000000, -1.000000000000000000 ) ) ;
#13151=AXIS2_PLACEMENT_3D ( 'NONE', #16595, #2482, #936 ) ;
#13153=DIRECTION ( 'NONE',  ( -1.000000000000000000, 0.000000000000000000, 6.994638739193269649E-15 ) ) ;
#13169=ORIENTED_EDGE ( 'NONE', *, *, #15761, .F. ) ;
#13181=DIRECTION ( 'NONE',  ( 0.5000000000000039968, 0.8660254037844363761, -3.491481338843161754E-15 ) ) ;
#13183=AXIS2_PLACEMENT_3D ( 'NONE', #17415, #15670, #17315 ) ;
#13194=ORIENTED_EDGE ( 'NONE', *, *, #5302, .F. ) ;
#13202=DIRECTION ( 'NONE',  ( 1.000000000000000000, 0.000000000000000000, -6.994638739193269649E-15 ) ) ;
#13218=DIRECTION ( 'NONE',  ( -6.982962677686266711E-15, 0.000000000000000000, -1.000000000000000000 ) ) ;
#13231=CIRCLE ( 'NONE', #1824, 127.4413876050234649 ) ;
#13242=EDGE_LOOP ( 'NONE', ( #18460, #4036, #11509, #16964, #8220 ) ) ;
#13275=CARTESIAN_POINT ( 'NONE',  ( -36.71940246244744799, 108.6254278180370250, 14.88498244535570869 ) ) ;
#13277=CARTESIAN_POINT ( 'NONE',  ( 103.2967819461768073, 53.25886146954521649, 14.88498244535472992 ) ) ;
#13298=CARTESIAN_POINT ( 'NONE',  ( 113.3640620605769413, -25.59923667990641150, 14.88498244535466064 ) ) ;
#13299=CARTESIAN_POINT ( 'NONE',  ( 1.396592535537252080E-14, 0.000000000000000000, 127.7817459305202448 ) ) ;
#13300=DIRECTION ( 'NONE',  ( 6.982962677686266711E-15, 0.000000000000000000, 1.000000000000000000 ) ) ;
#13303=DIRECTION ( 'NONE',  ( 0.5000000000000039968, 0.8660254037844362651, -3.488064225688950243E-15 ) ) ;
#13313=CARTESIAN_POINT ( 'NONE',  ( -2.300765332208364988, -116.0870680293436408, 14.88498244535546711 ) ) ;
#13321=VECTOR ( 'NONE', #19521, 1000.000000000000000 ) ;
#13323=CARTESIAN_POINT ( 'NONE',  ( 113.5802308907677372, 8.308367629983374414, 39.88498244535465886 ) ) ;
#13333=EDGE_CURVE ( 'NONE', #16627, #7331, #1944, .T. ) ;
#13337=DIRECTION ( 'NONE',  ( 1.000000000000000000, 0.000000000000000000, -6.994638739193269649E-15 ) ) ;
#13342=DIRECTION ( 'NONE',  ( -1.000000000000000000, 0.000000000000000000, 6.969309079188926949E-15 ) ) ;
#13357=DIRECTION ( 'NONE',  ( -6.982962677686266711E-15, 0.000000000000000000, -1.000000000000000000 ) ) ;
#13369=CIRCLE ( 'NONE', #4568, 106.4288957539801146 ) ;
#13374=FACE_OUTER_BOUND ( 'NONE', #2614, .T. ) ;
#13383=FACE_OUTER_BOUND ( 'NONE', #19430, .T. ) ;
#13400=( LENGTH_UNIT ( ) NAMED_UNIT ( * ) SI_UNIT ( .MILLI., .METRE. ) );
#13403=ORIENTED_EDGE ( 'NONE', *, *, #12594, .T. ) ;
#13413=VERTEX_POINT ( 'NONE', #17992 ) ;
#13421=VECTOR ( 'NONE', #5844, 1000.000000000000000 ) ;
#13437=VECTOR ( 'NONE', #235, 1000.000000000000000 ) ;
#13453=VERTEX_POINT ( 'NONE', #3961 ) ;
#13458=EDGE_LOOP ( 'NONE', ( #8092, #4321, #15438, #19152, #11467, #5383 ) ) ;
#13462=DIRECTION ( 'NONE',  ( 1.000000000000000000, 0.000000000000000000, -6.977185866873308817E-15 ) ) ;
#13487=CYLINDRICAL_SURFACE ( 'NONE', #19585, 3.224098631618460331 ) ;
#13500=DIRECTION ( 'NONE',  ( 1.000000000000000000, 0.000000000000000000, 0.000000000000000000 ) ) ;
#13501=CARTESIAN_POINT ( 'NONE',  ( -109.5721339228237667, 31.03941509555038181, 14.88498244535621851 ) ) ;
#13507=CIRCLE ( 'NONE', #460, 3.224098631618453670 ) ;
#13514=ORIENTED_EDGE ( 'NONE', *, *, #15502, .F. ) ;
#13528=CARTESIAN_POINT ( 'NONE',  ( -23.23469325536272478, -13.41455640552162443, 14.88498244535561454 ) ) ;
#13552=UNCERTAINTY_MEASURE_WITH_UNIT (LENGTH_MEASURE( 1.000000000000000082E-05 ), #4370, 'distance_accuracy_value', 'NONE');
#13566=EDGE_LOOP ( 'NONE', ( #15175, #1136, #7478, #17894 ) ) ;
#13569=AXIS2_PLACEMENT_3D ( 'NONE', #18283, #12021, #4259 ) ;
#13574=VECTOR ( 'NONE', #6561, 1000.000000000000000 ) ;
#13584=AXIS2_PLACEMENT_3D ( 'NONE', #11784, #19670, #17658 ) ;
#13602=AXIS2_PLACEMENT_3D ( 'NONE', #9540, #17329, #6377 ) ;
#13620=AXIS2_PLACEMENT_3D ( 'NONE', #16238, #19499, #19310 ) ;
#13633=CARTESIAN_POINT ( 'NONE',  ( -49.59485801383840453, -102.5175491340983882, 39.88498244535580284 ) ) ;
#13642=EDGE_CURVE ( 'NONE', #10957, #16647, #17434, .T. ) ;
#13666=AXIS2_PLACEMENT_3D ( 'NONE', #19043, #11248, #5028 ) ;
#13674=FILL_AREA_STYLE ('',( #2948 ) ) ;
#13676=EDGE_LOOP ( 'NONE', ( #15570, #8977, #1045, #15204, #11550 ) ) ;
#13679=VERTEX_POINT ( 'NONE', #12027 ) ;
#13683=LINE ( 'NONE', #4380, #14212 ) ;
#13685=CARTESIAN_POINT ( 'NONE',  ( 70.38703763562273252, -92.47916748300480094, 14.88498244535495907 ) ) ;
#13689=FACE_OUTER_BOUND ( 'NONE', #8194, .T. ) ;
#13691=ORIENTED_EDGE ( 'NONE', *, *, #7366, .T. ) ;
#13707=ADVANCED_FACE ( 'NONE', ( #2738 ), #19009, .T. ) ;
#13717=EDGE_LOOP ( 'NONE', ( #12161, #10292, #15423, #66 ) ) ;
#13724=DIRECTION ( 'NONE',  ( 0.000000000000000000, 0.000000000000000000, 1.000000000000000000 ) ) ;
#13789=FACE_OUTER_BOUND ( 'NONE', #8645, .T. ) ;
#13822=ORIENTED_EDGE ( 'NONE', *, *, #11209, .T. ) ;
#13833=ORIENTED_EDGE ( 'NONE', *, *, #1304, .T. ) ;
#13853=VECTOR ( 'NONE', #2513, 1000.000000000000000 ) ;
#13866=AXIS2_PLACEMENT_3D ( 'NONE', #17386, #16049, #9598 ) ;
#13867=CARTESIAN_POINT ( 'NONE',  ( -9.176097008933940202, -25.21111933077039069, 39.88498244535551862 ) ) ;
#13889=LINE ( 'NONE', #9080, #7338 ) ;
#13893=DIRECTION ( 'NONE',  ( -0.1736481776669273336, 0.9848077530122086864, 1.229460064647279041E-15 ) ) ;
#13924=AXIS2_PLACEMENT_3D ( 'NONE', #16549, #2632, #8856 ) ;
#13958=CARTESIAN_POINT ( 'NONE',  ( 92.34802049131684498, -66.64338626758360817, 14.88498244535480630 ) ) ;
#13972=ORIENTED_EDGE ( 'NONE', *, *, #5362, .T. ) ;
#13982=SURFACE_STYLE_USAGE ( .BOTH. , #11923 ) ;
#13991=EDGE_CURVE ( 'NONE', #7509, #19500, #1079, .T. ) ;
#14015=CIRCLE ( 'NONE', #5213, 3.224098631618455890 ) ;
#14024=ADVANCED_FACE ( 'NONE', ( #18569 ), #10783, .T. ) ;
#14036=DIRECTION ( 'NONE',  ( -1.000000000000000000, 0.000000000000000000, 7.137148015447434001E-15 ) ) ;
#14039=ORIENTED_EDGE ( 'NONE', *, *, #4401, .F. ) ;
#14055=CARTESIAN_POINT ( 'NONE',  ( -3.143238168843473623, 31.03941509555038181, 39.88498244535548309 ) ) ;
#14070=FACE_OUTER_BOUND ( 'NONE', #2532, .T. ) ;
#14096=CYLINDRICAL_SURFACE ( 'NONE', #15856, 3.224098631618460331 ) ;
#14101=ADVANCED_FACE ( 'NONE', ( #16316 ), #19476, .F. ) ;
#14137=EDGE_LOOP ( 'NONE', ( #4967, #18543, #1506, #3339 ) ) ;
#14138=EDGE_CURVE ( 'NONE', #6223, #2409, #7298, .T. ) ;
#14141=CARTESIAN_POINT ( 'NONE',  ( -109.5721339228237667, 31.03941509555038181, 14.88498244535621851 ) ) ;
#14146=CYLINDRICAL_SURFACE ( 'NONE', #12278, 106.4288957539801004 ) ;
#14162=APPLICATION_CONTEXT ( 'automotive_design' ) ;
#14168=EDGE_CURVE ( 'NONE', #18511, #19007, #10559, .T. ) ;
#14174=ADVANCED_FACE ( 'NONE', ( #5762 ), #7096, .T. ) ;
#14181=VERTEX_POINT ( 'NONE', #11978 ) ;
#14212=VECTOR ( 'NONE', #19926, 1000.000000000000000 ) ;
#14213=ORIENTED_EDGE ( 'NONE', *, *, #8482, .F. ) ;
#14216=ORIENTED_EDGE ( 'NONE', *, *, #6731, .F. ) ;
#14246=CARTESIAN_POINT ( 'NONE',  ( 1.396592535537252080E-14, 0.000000000000000000, 43.88498244535546178 ) ) ;
#14251=AXIS2_PLACEMENT_3D ( 'NONE', #4767, #15912, #5075 ) ;
#14262=EDGE_CURVE ( 'NONE', #7038, #18698, #17107, .T. ) ;
#14269=CIRCLE ( 'NONE', #11319, 3.224098631618453670 ) ;
#14284=EDGE_CURVE ( 'NONE', #1745, #11508, #20050, .T. ) ;
#14296=CARTESIAN_POINT ( 'NONE',  ( 26.85905058935142975, 1.464553941565464035, 14.88498244535526460 ) ) ;
#14339=DIRECTION ( 'NONE',  ( 6.982962677686266711E-15, -0.000000000000000000, 1.000000000000000000 ) ) ;
#14340=CARTESIAN_POINT ( 'NONE',  ( 100.5989061668484226, 55.02415981988612970, 39.88498244535475123 ) ) ;
#14383=ORIENTED_EDGE ( 'NONE', *, *, #3002, .T. ) ;
#14390=VERTEX_POINT ( 'NONE', #1671 ) ;
#14393=CARTESIAN_POINT ( 'NONE',  ( -17.24542129382122724, 20.55229278271246329, 14.88498244535557369 ) ) ;
#14408=LINE ( 'NONE', #9599, #16579 ) ;
#14409=FACE_OUTER_BOUND ( 'NONE', #6300, .T. ) ;
#14412=AXIS2_PLACEMENT_3D ( 'NONE', #3036, #4774, #18474 ) ;
#14416=ORIENTED_EDGE ( 'NONE', *, *, #6731, .T. ) ;
#14418=ORIENTED_EDGE ( 'NONE', *, *, #12485, .T. ) ;
#14437=DIRECTION ( 'NONE',  ( -1.000000000000000000, 0.000000000000000000, 6.976128451377902853E-15 ) ) ;
#14455=CARTESIAN_POINT ( 'NONE',  ( -5.951998377315654842, -25.21111933077039069, 14.88498244535549198 ) ) ;
#14468=AXIS2_PLACEMENT_3D ( 'NONE', #14757, #19370, #8617 ) ;
#14477=CARTESIAN_POINT ( 'NONE',  ( 113.3640620605771261, -25.59923667990641150, 39.88498244535465886 ) ) ;
#14484=EDGE_CURVE ( 'NONE', #10450, #8591, #5047, .T. ) ;
#14486=EDGE_LOOP ( 'NONE', ( #5215, #4243, #8337, #13972 ) ) ;
#14489=EDGE_CURVE ( 'NONE', #2170, #19703, #13507, .T. ) ;
#14496=VECTOR ( 'NONE', #14619, 1000.000000000000000 ) ;
#14504=DIRECTION ( 'NONE',  ( -6.982962677686265922E-15, -3.944304526105059903E-31, -1.000000000000000000 ) ) ;
#14509=DIRECTION ( 'NONE',  ( 6.982962677686266711E-15, -0.000000000000000000, 1.000000000000000000 ) ) ;
#14523=DIRECTION ( 'NONE',  ( 6.982962677686266711E-15, -0.000000000000000000, 1.000000000000000000 ) ) ;
#14531=DIRECTION ( 'NONE',  ( 1.000000000000000000, 0.000000000000000000, -6.994638739193269649E-15 ) ) ;
#14540=CIRCLE ( 'NONE', #13866, 3.224098631618458999 ) ;
#14551=CYLINDRICAL_SURFACE ( 'NONE', #5739, 3.224098631618460331 ) ;
#14554=ORIENTED_EDGE ( 'NONE', *, *, #7603, .F. ) ;
#14563=ORIENTED_EDGE ( 'NONE', *, *, #19701, .T. ) ;
#14567=ORIENTED_EDGE ( 'NONE', *, *, #12485, .F. ) ;
#14576=CIRCLE ( 'NONE', #533, 106.4288957539801004 ) ;
#14581=CARTESIAN_POINT ( 'NONE',  ( -20.01059462374409037, -13.41455640552162443, 39.88498244535559678 ) ) ;
#14589=AXIS2_PLACEMENT_3D ( 'NONE', #5086, #15922, #5187 ) ;
#14590=ORIENTED_EDGE ( 'NONE', *, *, #19867, .T. ) ;
#14596=DIRECTION ( 'NONE',  ( 6.982962677686266711E-15, -0.000000000000000000, 1.000000000000000000 ) ) ;
#14619=DIRECTION ( 'NONE',  ( -0.000000000000000000, -0.000000000000000000, -1.000000000000000000 ) ) ;
#14630=CYLINDRICAL_SURFACE ( 'NONE', #9054, 3.224098631618460331 ) ;
#14638=ORIENTED_EDGE ( 'NONE', *, *, #16313, .T. ) ;
#14639=ORIENTED_EDGE ( 'NONE', *, *, #2050, .T. ) ;
#14653=EDGE_CURVE ( 'NONE', #19558, #7864, #3077, .T. ) ;
#14661=CARTESIAN_POINT ( 'NONE',  ( 26.42151830275484770, 4.658826548058130790, 14.88498244535526815 ) ) ;
#14662=AXIS2_PLACEMENT_3D ( 'NONE', #12547, #18809, #9488 ) ;
#14667=VERTEX_POINT ( 'NONE', #11673 ) ;
#14676=CARTESIAN_POINT ( 'NONE',  ( -3.221721112346448201, 26.95290724009910832, 39.88498244535547599 ) ) ;
#14678=CIRCLE ( 'NONE', #6195, 3.224098631618460775 ) ;
#14696=FACE_OUTER_BOUND ( 'NONE', #12232, .T. ) ;
#14703=DIRECTION ( 'NONE',  ( 0.9396926207859057634, -0.3420201433256758183, -6.456589605409169860E-15 ) ) ;
#14713=AXIS2_PLACEMENT_3D ( 'NONE', #5254, #17731, #8514 ) ;
#14716=CARTESIAN_POINT ( 'NONE',  ( 48.09719419928514128, 107.5784105627835174, 39.88498244535512072 ) ) ;
#14717=CARTESIAN_POINT ( 'NONE',  ( 1.396592535537253342E-14, 0.000000000000000000, 43.88498244535545467 ) ) ;
#14721=ADVANCED_FACE ( 'NONE', ( #15047 ), #10329, .T. ) ;
#14730=DIRECTION ( 'NONE',  ( -0.7660444431189857850, -0.6427876096865299260, 5.349259755748838558E-15 ) ) ;
#14739=EDGE_CURVE ( 'NONE', #6064, #6223, #1777, .T. ) ;
#14751=CARTESIAN_POINT ( 'NONE',  ( -82.43884259638412004, -58.61746404108814801, 14.88498244535602844 ) ) ;
#14754=CARTESIAN_POINT ( 'NONE',  ( 105.9946577255055331, 51.49356311920430329, 39.88498244535471571 ) ) ;
#14756=CYLINDRICAL_SURFACE ( 'NONE', #5811, 3.224098631618460331 ) ;
#14757=CARTESIAN_POINT ( 'NONE',  ( -17.24542129382122724, 20.55229278271246329, 14.88498244535557369 ) ) ;
#14765=CARTESIAN_POINT ( 'NONE',  ( 1.396592535537252080E-14, 0.000000000000000000, 43.88498244535546178 ) ) ;
#14769=EDGE_CURVE ( 'NONE', #11267, #17576, #19735, .T. ) ;
#14773=FACE_OUTER_BOUND ( 'NONE', #18754, .T. ) ;
#14778=EDGE_LOOP ( 'NONE', ( #11440, #11092 ) ) ;
#14784=AXIS2_PLACEMENT_3D ( 'NONE', #16589, #12274, #15144 ) ;
#14791=EDGE_CURVE ( 'NONE', #13413, #807, #7648, .T. ) ;
#14814=DIRECTION ( 'NONE',  ( -6.982962677686266711E-15, 0.000000000000000000, -1.000000000000000000 ) ) ;
#14826=CARTESIAN_POINT ( 'NONE',  ( -78.85162031257850401, -85.37653928070189124, 14.88498244535600357 ) ) ;
#14831=CYLINDRICAL_SURFACE ( 'NONE', #12190, 106.4288957539801004 ) ;
#14832=ORIENTED_EDGE ( 'NONE', *, *, #17165, .F. ) ;
#14836=DIRECTION ( 'NONE',  ( -6.982962677686266711E-15, 0.000000000000000000, -1.000000000000000000 ) ) ;
#14846=AXIS2_PLACEMENT_3D ( 'NONE', #19047, #1956, #8184 ) ;
#14849=EDGE_LOOP ( 'NONE', ( #17057, #7324, #10135, #17453 ) ) ;
#14860=AXIS2_PLACEMENT_3D ( 'NONE', #1003, #2652, #2259 ) ;
#14864=CARTESIAN_POINT ( 'NONE',  ( 73.61113626724119285, -92.47916748300480094, 14.88498244535493598 ) ) ;
#14879=EDGE_CURVE ( 'NONE', #15471, #12923, #8643, .T. ) ;
#14892=EDGE_CURVE ( 'NONE', #17841, #19981, #2115, .T. ) ;
#14899=DIRECTION ( 'NONE',  ( -6.982962677686266711E-15, 0.000000000000000000, -1.000000000000000000 ) ) ;
#14919=CARTESIAN_POINT ( 'NONE',  ( 92.34802049131684498, -66.64338626758360817, 14.88498244535480630 ) ) ;
#14921=CARTESIAN_POINT ( 'NONE',  ( -115.2828271789296650, -14.71737894807794156, 14.88498244535625759 ) ) ;
#14936=AXIS2_PLACEMENT_3D ( 'NONE', #5921, #8868, #3054 ) ;
#14966=AXIS2_PLACEMENT_3D ( 'NONE', #797, #14814, #7241 ) ;
#14973=ORIENTED_EDGE ( 'NONE', *, *, #9610, .F. ) ;
#14978=ORIENTED_EDGE ( 'NONE', *, *, #2251, .T. ) ;
#14983=AXIS2_PLACEMENT_3D ( 'NONE', #2027, #19112, #5297 ) ;
#14990=FACE_OUTER_BOUND ( 'NONE', #528, .T. ) ;
#15022=CYLINDRICAL_SURFACE ( 'NONE', #14860, 106.4288957539801004 ) ;
#15023=ORIENTED_EDGE ( 'NONE', *, *, #8219, .T. ) ;
#15028=ORIENTED_EDGE ( 'NONE', *, *, #20238, .F. ) ;
#15030=CARTESIAN_POINT ( 'NONE',  ( 114.2960429025576587, -28.68569479505797659, 14.88498244535465354 ) ) ;
#15031=DIRECTION ( 'NONE',  ( 6.982962677686266711E-15, -0.000000000000000000, 1.000000000000000000 ) ) ;
#15032=ORIENTED_EDGE ( 'NONE', *, *, #15121, .F. ) ;
#15047=FACE_OUTER_BOUND ( 'NONE', #17470, .T. ) ;
#15057=VERTEX_POINT ( 'NONE', #19625 ) ;
#15071=LINE ( 'NONE', #8731, #236 ) ;
#15086=VERTEX_POINT ( 'NONE', #10023 ) ;
#15088=DIRECTION ( 'NONE',  ( -0.7660444431189862291, -0.6427876096865298150, 4.304393070272780959E-15 ) ) ;
#15091=ADVANCED_FACE ( 'NONE', ( #8783 ), #15022, .F. ) ;
#15097=DIRECTION ( 'NONE',  ( 6.982962677686266711E-15, -0.000000000000000000, 1.000000000000000000 ) ) ;
#15105=CIRCLE ( 'NONE', #4332, 112.8770930172170210 ) ;
#15111=CARTESIAN_POINT ( 'NONE',  ( 1.396592535537252080E-14, 0.000000000000000000, 49.99999999999998579 ) ) ;
#15121=EDGE_CURVE ( 'NONE', #1501, #1401, #18123, .T. ) ;
#15130=ORIENTED_EDGE ( 'NONE', *, *, #19993, .T. ) ;
#15132=AXIS2_PLACEMENT_3D ( 'NONE', #3068, #9302, #6139 ) ;
#15137=EDGE_LOOP ( 'NONE', ( #11947, #2213 ) ) ;
#15143=DIRECTION ( 'NONE',  ( -6.982962677686266711E-15, 0.000000000000000000, -1.000000000000000000 ) ) ;
#15144=DIRECTION ( 'NONE',  ( 1.000000000000000000, 0.000000000000000000, -6.976128451377903642E-15 ) ) ;
#15175=ORIENTED_EDGE ( 'NONE', *, *, #5861, .T. ) ;
#15176=CARTESIAN_POINT ( 'NONE',  ( -9.176097008934114285, -25.21111933077039069, 14.88498244535551507 ) ) ;
#15178=EDGE_LOOP ( 'NONE', ( #5883, #16430, #18541, #5240 ) ) ;
#15186=ORIENTED_EDGE ( 'NONE', *, *, #10096, .F. ) ;
#15190=EDGE_LOOP ( 'NONE', ( #7316, #9041, #7482, #11589 ) ) ;
#15193=CARTESIAN_POINT ( 'NONE',  ( -3.221721112346616067, 26.95290724009910832, 14.88498244535547244 ) ) ;
#15204=ORIENTED_EDGE ( 'NONE', *, *, #6618, .T. ) ;
#15216=CIRCLE ( 'NONE', #16177, 3.224098631618460775 ) ;
#15224=FACE_BOUND ( 'NONE', #4450, .T. ) ;
#15238=CARTESIAN_POINT ( 'NONE',  ( -9.176097008934114285, -25.21111933077039069, 14.88498244535551507 ) ) ;
#15239=EDGE_CURVE ( 'NONE', #17104, #18698, #13889, .T. ) ;
#15245=CARTESIAN_POINT ( 'NONE',  ( -25.74015858913164578, 7.810105800529631992, 14.88498244535563231 ) ) ;
#15250=FACE_OUTER_BOUND ( 'NONE', #14486, .T. ) ;
#15257=EDGE_CURVE ( 'NONE', #19127, #11748, #13683, .T. ) ;
#15283=ADVANCED_BREP_SHAPE_REPRESENTATION ( '', ( #1084, #18639 ), #4580 ) ;
#15293=ADVANCED_FACE ( 'NONE', ( #12557 ), #14096, .T. ) ;
#15321=DIRECTION ( 'NONE',  ( 6.982962677686266711E-15, -0.000000000000000000, 1.000000000000000000 ) ) ;
#15329=FACE_BOUND ( 'NONE', #17343, .T. ) ;
#15336=CIRCLE ( 'NONE', #16002, 106.4288957539801004 ) ;
#15339=ORIENTED_EDGE ( 'NONE', *, *, #14489, .F. ) ;
#15372=FACE_OUTER_BOUND ( 'NONE', #14137, .T. ) ;
#15373=ORIENTED_EDGE ( 'NONE', *, *, #12348, .T. ) ;
#15374=DIRECTION ( 'NONE',  ( 0.9396926207859063185, -0.3420201433256742640, -6.456589605409180904E-15 ) ) ;
#15389=EDGE_LOOP ( 'NONE', ( #19475, #17060, #792, #5582 ) ) ;
#15409=ORIENTED_EDGE ( 'NONE', *, *, #19509, .T. ) ;
#15411=CARTESIAN_POINT ( 'NONE',  ( 42.44352287704968063, 94.20918150411493741, 14.88498244535515624 ) ) ;
#15413=EDGE_CURVE ( 'NONE', #2014, #9259, #14540, .T. ) ;
#15422=DIRECTION ( 'NONE',  ( 1.000000000000000000, 0.000000000000000000, -6.977185866873308817E-15 ) ) ;
#15423=ORIENTED_EDGE ( 'NONE', *, *, #11773, .F. ) ;
#15426=ORIENTED_EDGE ( 'NONE', *, *, #5405, .T. ) ;
#15431=AXIS2_PLACEMENT_3D ( 'NONE', #735, #6792, #16200 ) ;
#15438=ORIENTED_EDGE ( 'NONE', *, *, #18017, .F. ) ;
#15439=AXIS2_PLACEMENT_3D ( 'NONE', #19827, #1008, #14730 ) ;
#15440=CIRCLE ( 'NONE', #9231, 3.224098631618460331 ) ;
#15452=DIRECTION ( 'NONE',  ( -0.1736481776669408228, -0.9848077530122062440, 2.152196535136390085E-15 ) ) ;
#15462=VECTOR ( 'NONE', #16193, 1000.000000000000000 ) ;
#15471=VERTEX_POINT ( 'NONE', #6337 ) ;
#15486=CARTESIAN_POINT ( 'NONE',  ( -63.98537287693041264, 94.20918150411493741, 14.88498244535589876 ) ) ;
#15497=CARTESIAN_POINT ( 'NONE',  ( -8.402595070145098433, -117.5408478153264298, 14.88498244535551152 ) ) ;
#15502=EDGE_CURVE ( 'NONE', #1080, #13413, #16183, .T. ) ;
#15541=DIRECTION ( 'NONE',  ( 1.000000000000000000, 0.000000000000000000, -6.994638739193269649E-15 ) ) ;
#15546=VERTEX_POINT ( 'NONE', #14754 ) ;
#15559=DIRECTION ( 'NONE',  ( -6.982962677686266711E-15, 0.000000000000000000, -1.000000000000000000 ) ) ;
#15566=ORIENTED_EDGE ( 'NONE', *, *, #6535, .F. ) ;
#15570=ORIENTED_EDGE ( 'NONE', *, *, #14739, .T. ) ;
#15579=DIRECTION ( 'NONE',  ( 6.982962677686266711E-15, -0.000000000000000000, 1.000000000000000000 ) ) ;
#15580=CARTESIAN_POINT ( 'NONE',  ( -26.42151830275497915, 4.658826548058537576, 39.88498244535563941 ) ) ;
#15591=FACE_OUTER_BOUND ( 'NONE', #2220, .T. ) ;
#15595=EDGE_CURVE ( 'NONE', #2786, #17433, #10945, .T. ) ;
#15611=DIRECTION ( 'NONE',  ( -0.7660444431189862291, -0.6427876096865298150, 5.380491337840976593E-15 ) ) ;
#15630=AXIS2_PLACEMENT_3D ( 'NONE', #15976, #8291, #4941 ) ;
#15632=CARTESIAN_POINT ( 'NONE',  ( -109.5721339228237667, 31.03941509555038181, 14.88498244535621851 ) ) ;
#15651=ORIENTED_EDGE ( 'NONE', *, *, #5782, .F. ) ;
#15664=EDGE_CURVE ( 'NONE', #10905, #2341, #19764, .T. ) ;
#15665=CARTESIAN_POINT ( 'NONE',  ( -103.8888757476053541, -46.65403860089418941, 14.88498244535617765 ) ) ;
#15670=DIRECTION ( 'NONE',  ( 6.982962677686266711E-15, -0.000000000000000000, 1.000000000000000000 ) ) ;
#15675=EDGE_CURVE ( 'NONE', #3202, #17939, #18722, .T. ) ;
#15714=LINE ( 'NONE', #1696, #10461 ) ;
#15731=EDGE_LOOP ( 'NONE', ( #5102, #17962, #619, #17743 ) ) ;
#15747=ORIENTED_EDGE ( 'NONE', *, *, #15413, .T. ) ;
#15761=EDGE_CURVE ( 'NONE', #10905, #16353, #16692, .T. ) ;
#15762=DIRECTION ( 'NONE',  ( 1.000000000000000000, 0.000000000000000000, -6.976128451377902853E-15 ) ) ;
#15775=EDGE_CURVE ( 'NONE', #6744, #1994, #7186, .T. ) ;
#15779=CARTESIAN_POINT ( 'NONE',  ( -1.396592535537253342E-14, 0.000000000000000000, 39.88498244535545467 ) ) ;
#15790=ADVANCED_FACE ( 'NONE', ( #12065 ), #16592, .T. ) ;
#15825=ORIENTED_EDGE ( 'NONE', *, *, #4242, .F. ) ;
#15832=FACE_OUTER_BOUND ( 'NONE', #15988, .T. ) ;
#15853=ORIENTED_EDGE ( 'NONE', *, *, #15595, .F. ) ;
#15856=AXIS2_PLACEMENT_3D ( 'NONE', #5006, #2034, #3564 ) ;
#15872=DIRECTION ( 'NONE',  ( -6.982962677686266711E-15, 0.000000000000000000, -1.000000000000000000 ) ) ;
#15889=CARTESIAN_POINT ( 'NONE',  ( -109.5721339228235820, 31.03941509555038181, 39.88498244535622206 ) ) ;
#15891=CIRCLE ( 'NONE', #5435, 106.4288957539801288 ) ;
#15905=EDGE_CURVE ( 'NONE', #18684, #4108, #11185, .T. ) ;
#15912=DIRECTION ( 'NONE',  ( 6.982962677686266711E-15, 0.000000000000000000, 1.000000000000000000 ) ) ;
#15919=DIRECTION ( 'NONE',  ( -6.982962677686266711E-15, 0.000000000000000000, -1.000000000000000000 ) ) ;
#15922=DIRECTION ( 'NONE',  ( -6.982962677686266711E-15, 0.000000000000000000, -1.000000000000000000 ) ) ;
#15924=AXIS2_PLACEMENT_3D ( 'NONE', #19221, #19319, #16147 ) ;
#15925=ORIENTED_EDGE ( 'NONE', *, *, #11507, .F. ) ;
#15943=PLANE ( 'NONE',  #8465 ) ;
#15944=CARTESIAN_POINT ( 'NONE',  ( -75.71267875615008336, -86.11264925328200093, 39.88498244535598047 ) ) ;
#15974=DIRECTION ( 'NONE',  ( 6.982962677686266711E-15, -0.000000000000000000, 1.000000000000000000 ) ) ;
#15976=CARTESIAN_POINT ( 'NONE',  ( -109.5721339228237667, 31.03941509555038181, 14.88498244535621851 ) ) ;
#15978=EDGE_LOOP ( 'NONE', ( #7640, #11565, #4089, #7541 ) ) ;
#15988=EDGE_LOOP ( 'NONE', ( #5043, #19811, #5306, #7351 ) ) ;
#15995=ADVANCED_FACE ( 'NONE', ( #3888 ), #2356, .T. ) ;
#15997=EDGE_CURVE ( 'NONE', #7864, #15086, #1056, .T. ) ;
#16002=AXIS2_PLACEMENT_3D ( 'NONE', #13958, #18785, #2823 ) ;
#16020=LINE ( 'NONE', #1898, #20236 ) ;
#16036=DIRECTION ( 'NONE',  ( 6.982962677686266711E-15, -0.000000000000000000, 1.000000000000000000 ) ) ;
#16049=DIRECTION ( 'NONE',  ( -6.982962677686266711E-15, 0.000000000000000000, -1.000000000000000000 ) ) ;
#16053=ADVANCED_FACE ( 'NONE', ( #4180 ), #10413, .F. ) ;
#16090=CARTESIAN_POINT ( 'NONE',  ( -117.2142335457655520, -12.13581325405623268, 14.88498244535627002 ) ) ;
#16107=EDGE_CURVE ( 'NONE', #15546, #12565, #15105, .T. ) ;
#16113=VECTOR ( 'NONE', #10025, 1000.000000000000000 ) ;
#16125=ORIENTED_EDGE ( 'NONE', *, *, #14892, .F. ) ;
#16138=CARTESIAN_POINT ( 'NONE',  ( 27.90514497005375461, -110.4119590718113244, 14.88498244535525750 ) ) ;
#16147=DIRECTION ( 'NONE',  ( -0.7660444431189770143, 0.6427876096865404731, 5.346191897317644012E-15 ) ) ;
#16155=VERTEX_POINT ( 'NONE', #8263 ) ;
#16177=AXIS2_PLACEMENT_3D ( 'NONE', #15580, #5057, #131 ) ;
#16181=DIRECTION ( 'NONE',  ( 1.000000000000000000, 0.000000000000000000, -6.976128451377902853E-15 ) ) ;
#16183=CIRCLE ( 'NONE', #9962, 106.4288957539801146 ) ;
#16188=EDGE_CURVE ( 'NONE', #2555, #2184, #8058, .T. ) ;
#16189=ORIENTED_EDGE ( 'NONE', *, *, #16491, .F. ) ;
#16192=CIRCLE ( 'NONE', #1814, 127.4413876050234649 ) ;
#16193=DIRECTION ( 'NONE',  ( 6.982962677686266711E-15, -0.000000000000000000, 1.000000000000000000 ) ) ;
#16197=EDGE_CURVE ( 'NONE', #17104, #2440, #4125, .T. ) ;
#16200=DIRECTION ( 'NONE',  ( 1.000000000000000000, 0.000000000000000000, -6.994638739193269649E-15 ) ) ;
#16222=DIRECTION ( 'NONE',  ( -1.000000000000000000, 0.000000000000000000, 6.982962677686266711E-15 ) ) ;
#16238=CARTESIAN_POINT ( 'NONE',  ( 17.24542129382117750, 20.55229278271219329, 14.88498244535533033 ) ) ;
#16251=EDGE_CURVE ( 'NONE', #2918, #12798, #10662, .T. ) ;
#16253=DIRECTION ( 'NONE',  ( 0.4999999999999918954, -0.8660254037844433705, -3.503961184244745387E-15 ) ) ;
#16281=EDGE_CURVE ( 'NONE', #2426, #17841, #14269, .T. ) ;
#16291=ORIENTED_EDGE ( 'NONE', *, *, #18793, .T. ) ;
#16298=CIRCLE ( 'NONE', #17912, 127.4413876050234649 ) ;
#16303=ADVANCED_FACE ( 'NONE', ( #5594 ), #10291, .T. ) ;
#16313=EDGE_CURVE ( 'NONE', #9831, #18511, #2334, .T. ) ;
#16316=FACE_OUTER_BOUND ( 'NONE', #6890, .T. ) ;
#16330=AXIS2_PLACEMENT_3D ( 'NONE', #1384, #17044, #3224 ) ;
#16331=ORIENTED_EDGE ( 'NONE', *, *, #19716, .F. ) ;
#16342=DIRECTION ( 'NONE',  ( 1.000000000000000000, 0.000000000000000000, -7.137148015447434001E-15 ) ) ;
#16353=VERTEX_POINT ( 'NONE', #9058 ) ;
#16382=ORIENTED_EDGE ( 'NONE', *, *, #4869, .F. ) ;
#16386=EDGE_CURVE ( 'NONE', #16400, #3088, #18852, .T. ) ;
#16390=CIRCLE ( 'NONE', #7219, 17.50000000000000355 ) ;
#16400=VERTEX_POINT ( 'NONE', #12325 ) ;
#16405=AXIS2_PLACEMENT_3D ( 'NONE', #6310, #12427, #12317 ) ;
#16430=ORIENTED_EDGE ( 'NONE', *, *, #19701, .F. ) ;
#16435=ORIENTED_EDGE ( 'NONE', *, *, #15997, .F. ) ;
#16436=CARTESIAN_POINT ( 'NONE',  ( 17.24542129382117750, 20.55229278271219329, 14.88498244535533033 ) ) ;
#16444=ORIENTED_EDGE ( 'NONE', *, *, #9144, .T. ) ;
#16451=CARTESIAN_POINT ( 'NONE',  ( 112.4320812185964371, -22.51277856475483574, 39.88498244535466597 ) ) ;
#16452=DIRECTION ( 'NONE',  ( 0.4999999999999916178, -0.8660254037844435926, -4.304393070272782536E-15 ) ) ;
#16483=ORIENTED_EDGE ( 'NONE', *, *, #18991, .F. ) ;
#16488=ORIENTED_EDGE ( 'NONE', *, *, #19520, .T. ) ;
#16491=EDGE_CURVE ( 'NONE', #4614, #8547, #3165, .T. ) ;
#16501=ADVANCED_FACE ( 'NONE', ( #11101 ), #3337, .T. ) ;
#16520=DIRECTION ( 'NONE',  ( -0.1736481776669408228, -0.9848077530122062440, 1.076098267568195042E-15 ) ) ;
#16535=LINE ( 'NONE', #10278, #13853 ) ;
#16549=CARTESIAN_POINT ( 'NONE',  ( 1.396592535537252080E-14, 0.000000000000000000, 49.99999999999998579 ) ) ;
#16551=AXIS2_PLACEMENT_3D ( 'NONE', #17787, #5698, #3954 ) ;
#16553=ORIENTED_EDGE ( 'NONE', *, *, #1543, .F. ) ;
#16571=FACE_OUTER_BOUND ( 'NONE', #18650, .T. ) ;
#16579=VECTOR ( 'NONE', #7957, 1000.000000000000000 ) ;
#16581=DIRECTION ( 'NONE',  ( -6.982962677686266711E-15, 0.000000000000000000, -1.000000000000000000 ) ) ;
#16583=ORIENTED_EDGE ( 'NONE', *, *, #14138, .F. ) ;
#16589=CARTESIAN_POINT ( 'NONE',  ( 81.66698895276879000, 79.37254397626031732, 14.88498244535488269 ) ) ;
#16592=CYLINDRICAL_SURFACE ( 'NONE', #18391, 3.224098631618460331 ) ;
#16594=DIRECTION ( 'NONE',  ( -6.982962677686266711E-15, 0.000000000000000000, -1.000000000000000000 ) ) ;
#16595=CARTESIAN_POINT ( 'NONE',  ( -63.98537287693041264, 94.20918150411493741, 14.88498244535589876 ) ) ;
#16600=AXIS2_PLACEMENT_3D ( 'NONE', #1209, #12150, #18411 ) ;
#16605=FACE_OUTER_BOUND ( 'NONE', #19957, .T. ) ;
#16606=CARTESIAN_POINT ( 'NONE',  ( -25.74015858913164578, 7.810105800529631992, 14.88498244535563231 ) ) ;
#16618=DIRECTION ( 'NONE',  ( 1.000000000000000000, 0.000000000000000000, -6.994638739193269649E-15 ) ) ;
#16623=AXIS2_PLACEMENT_3D ( 'NONE', #7922, #10991, #3227 ) ;
#16627=VERTEX_POINT ( 'NONE', #19951 ) ;
#16629=CIRCLE ( 'NONE', #8126, 106.4288957539800862 ) ;
#16636=DIRECTION ( 'NONE',  ( 6.982962677686266711E-15, -0.000000000000000000, 1.000000000000000000 ) ) ;
#16644=DIRECTION ( 'NONE',  ( -6.982962677686266711E-15, 0.000000000000000000, -1.000000000000000000 ) ) ;
#16647=VERTEX_POINT ( 'NONE', #10531 ) ;
#16670=CARTESIAN_POINT ( 'NONE',  ( 11.54085525628718401, 113.2974248684783163, 14.88498244535537296 ) ) ;
#16692=LINE ( 'NONE', #11768, #17414 ) ;
#16702=CARTESIAN_POINT ( 'NONE',  ( -127.4413876050234364, 1.560706874093891490E-14, 43.88498244535634285 ) ) ;
#16703=ORIENTED_EDGE ( 'NONE', *, *, #3905, .F. ) ;
#16751=EDGE_LOOP ( 'NONE', ( #2217, #20151, #3547, #2707 ) ) ;
#16758=CIRCLE ( 'NONE', #13151, 112.8770930172170495 ) ;
#16761=EDGE_LOOP ( 'NONE', ( #2368, #7308, #16125, #13822 ) ) ;
#16762=DIRECTION ( 'NONE',  ( 6.982962677686266711E-15, -0.000000000000000000, 1.000000000000000000 ) ) ;
#16774=EDGE_CURVE ( 'NONE', #17939, #14181, #1198, .T. ) ;
#16791=CARTESIAN_POINT ( 'NONE',  ( 26.42151830275484770, 4.658826548058130790, 14.88498244535526815 ) ) ;
#16797=AXIS2_PLACEMENT_3D ( 'NONE', #14246, #15579, #7585 ) ;
#16801=EDGE_CURVE ( 'NONE', #16155, #3088, #6669, .T. ) ;
#16805=DIRECTION ( 'NONE',  ( 0.5000000000000044409, 0.8660254037844360431, -4.304393070272782536E-15 ) ) ;
#16806=DIRECTION ( 'NONE',  ( 1.000000000000000000, 0.000000000000000000, -6.976128451377902853E-15 ) ) ;
#16830=CIRCLE ( 'NONE', #7043, 3.224098631618461663 ) ;
#16841=ORIENTED_EDGE ( 'NONE', *, *, #478, .F. ) ;
#16843=CARTESIAN_POINT ( 'NONE',  ( 113.5802308907675666, 8.308367629983374414, 14.88498244535465709 ) ) ;
#16855=CARTESIAN_POINT ( 'NONE',  ( -5.524863963826822655, -116.0870680293436408, 14.88498244535549020 ) ) ;
#16860=CARTESIAN_POINT ( 'NONE',  ( 73.61113626724119285, -92.47916748300480094, 14.88498244535493598 ) ) ;
#16896=CARTESIAN_POINT ( 'NONE',  ( -9.176097008934114285, -25.21111933077039069, 14.88498244535551507 ) ) ;
#16902=VERTEX_POINT ( 'NONE', #13275 ) ;
#16922=ADVANCED_FACE ( 'NONE', ( #16571 ), #3782, .T. ) ;
#16964=ORIENTED_EDGE ( 'NONE', *, *, #2727, .F. ) ;
#16965=CARTESIAN_POINT ( 'NONE',  ( -127.4413876050234933, 1.560706874093891806E-14, 39.88498244535634285 ) ) ;
#16973=DIRECTION ( 'NONE',  ( -6.982962677686266711E-15, 0.000000000000000000, -1.000000000000000000 ) ) ;
#16990=ADVANCED_FACE ( 'NONE', ( #2452 ), #14630, .T. ) ;
#16995=LINE ( 'NONE', #2982, #2385 ) ;
#16996=AXIS2_PLACEMENT_3D ( 'NONE', #13298, #7275, #2476 ) ;
#16999=CIRCLE ( 'NONE', #14713, 106.4288957539801004 ) ;
#17002=FACE_OUTER_BOUND ( 'NONE', #15978, .T. ) ;
#17005=ORIENTED_EDGE ( 'NONE', *, *, #14879, .T. ) ;
#17007=ADVANCED_FACE ( 'NONE', ( #19725 ), #7652, .T. ) ;
#17013=VECTOR ( 'NONE', #1743, 1000.000000000000000 ) ;
#17019=DIRECTION ( 'NONE',  ( -6.982962677686266711E-15, 0.000000000000000000, -1.000000000000000000 ) ) ;
#17024=LINE ( 'NONE', #9343, #12442 ) ;
#17025=DIRECTION ( 'NONE',  ( 6.982962677686266711E-15, -0.000000000000000000, 1.000000000000000000 ) ) ;
#17038=CARTESIAN_POINT ( 'NONE',  ( -9.544791666812290742, 100.7028639675991855, 14.88498244535551862 ) ) ;
#17044=DIRECTION ( 'NONE',  ( 6.982962677686266711E-15, -0.000000000000000000, 1.000000000000000000 ) ) ;
#17057=ORIENTED_EDGE ( 'NONE', *, *, #5782, .T. ) ;
#17060=ORIENTED_EDGE ( 'NONE', *, *, #13642, .F. ) ;
#17061=DIRECTION ( 'NONE',  ( 1.000000000000000000, 0.000000000000000000, -6.994638739193269649E-15 ) ) ;
#17064=SURFACE_STYLE_FILL_AREA ( #13674 ) ;
#17065=CARTESIAN_POINT ( 'NONE',  ( -103.8888757476053541, -46.65403860089418941, 14.88498244535617765 ) ) ;
#17067=FACE_OUTER_BOUND ( 'NONE', #9632, .T. ) ;
#17092=CARTESIAN_POINT ( 'NONE',  ( -115.2828271789294803, -14.71737894807794156, 39.88498244535625759 ) ) ;
#17099=ORIENTED_EDGE ( 'NONE', *, *, #13003, .T. ) ;
#17104=VERTEX_POINT ( 'NONE', #1316 ) ;
#17105=ORIENTED_EDGE ( 'NONE', *, *, #896, .T. ) ;
#17107=CIRCLE ( 'NONE', #16797, 27.50000000000000355 ) ;
#17128=CARTESIAN_POINT ( 'NONE',  ( 48.89172014028660129, 94.20918150411493741, 14.88498244535511184 ) ) ;
#17131=ADVANCED_FACE ( 'NONE', ( #13789 ), #18303, .T. ) ;
#17134=ORIENTED_EDGE ( 'NONE', *, *, #8028, .F. ) ;
#17149=DIRECTION ( 'NONE',  ( 6.982962677686266711E-15, -0.000000000000000000, 1.000000000000000000 ) ) ;
#17150=EDGE_CURVE ( 'NONE', #6726, #2555, #7111, .T. ) ;
#17151=CARTESIAN_POINT ( 'NONE',  ( 3.304959094393253416, 31.03941509555038181, 14.88498244535543158 ) ) ;
#17165=EDGE_CURVE ( 'NONE', #7250, #2555, #14408, .T. ) ;
#17180=EDGE_CURVE ( 'NONE', #2426, #2170, #11337, .T. ) ;
#17202=DIRECTION ( 'NONE',  ( -0.1736481776669409338, -0.9848077530122062440, 2.152196535136391268E-15 ) ) ;
#17203=ORIENTED_EDGE ( 'NONE', *, *, #14284, .T. ) ;
#17208=CIRCLE ( 'NONE', #14251, 106.4288957539801004 ) ;
#17242=ORIENTED_EDGE ( 'NONE', *, *, #2727, .T. ) ;
#17248=ORIENTED_EDGE ( 'NONE', *, *, #17180, .T. ) ;
#17253=CARTESIAN_POINT ( 'NONE',  ( -75.71267875615025389, -86.11264925328200093, 14.88498244535597870 ) ) ;
#17290=ORIENTED_EDGE ( 'NONE', *, *, #14739, .F. ) ;
#17295=DIRECTION ( 'NONE',  ( 6.982962677686266711E-15, -0.000000000000000000, 1.000000000000000000 ) ) ;
#17300=CARTESIAN_POINT ( 'NONE',  ( 113.5802308907675666, 8.308367629983374414, 14.88498244535465709 ) ) ;
#17313=APPLICATION_CONTEXT ( 'automotive_design' ) ;
#17315=DIRECTION ( 'NONE',  ( 1.000000000000000000, 0.000000000000000000, -6.976128451377902853E-15 ) ) ;
#17327=CARTESIAN_POINT ( 'NONE',  ( -25.74015858913147170, 7.810105800529631992, 39.88498244535563231 ) ) ;
#17329=DIRECTION ( 'NONE',  ( -6.982962677686266711E-15, 0.000000000000000000, -1.000000000000000000 ) ) ;
#17334=EDGE_CURVE ( 'NONE', #10728, #4820, #19834, .T. ) ;
#17341=LINE ( 'NONE', #8109, #1017 ) ;
#17343=EDGE_LOOP ( 'NONE', ( #6016, #10620, #13514, #9479, #4497 ) ) ;
#17363=EDGE_CURVE ( 'NONE', #13453, #9086, #5473, .T. ) ;
#17365=DIRECTION ( 'NONE',  ( -1.000000000000000000, 0.000000000000000000, 6.982962677686266711E-15 ) ) ;
#17371=ORIENTED_EDGE ( 'NONE', *, *, #3890, .T. ) ;
#17386=CARTESIAN_POINT ( 'NONE',  ( -115.2828271789296650, -14.71737894807794156, 14.88498244535625759 ) ) ;
#17414=VECTOR ( 'NONE', #5548, 1000.000000000000000 ) ;
#17415=CARTESIAN_POINT ( 'NONE',  ( -63.98537287693041264, 94.20918150411493741, 14.88498244535589876 ) ) ;
#17419=ORIENTED_EDGE ( 'NONE', *, *, #2251, .F. ) ;
#17420=EDGE_CURVE ( 'NONE', #16902, #1745, #1902, .T. ) ;
#17423=ORIENTED_EDGE ( 'NONE', *, *, #11873, .F. ) ;
#17424=ORIENTED_EDGE ( 'NONE', *, *, #19867, .F. ) ;
#17425=ORIENTED_EDGE ( 'NONE', *, *, #1891, .F. ) ;
#17433=VERTEX_POINT ( 'NONE', #16451 ) ;
#17434=CIRCLE ( 'NONE', #3369, 106.4288957539800862 ) ;
#17445=CARTESIAN_POINT ( 'NONE',  ( 0.000000000000000000, 0.000000000000000000, 49.99999999999999289 ) ) ;
#17453=ORIENTED_EDGE ( 'NONE', *, *, #11514, .T. ) ;
#17460=LINE ( 'NONE', #8329, #6939 ) ;
#17464=CARTESIAN_POINT ( 'NONE',  ( -49.59485801383840453, -102.5175491340983882, 39.88498244535580284 ) ) ;
#17465=ORIENTED_EDGE ( 'NONE', *, *, #2464, .T. ) ;
#17468=ORIENTED_EDGE ( 'NONE', *, *, #17150, .F. ) ;
#17470=EDGE_LOOP ( 'NONE', ( #15747, #4708, #18723, #7432, #9289 ) ) ;
#17474=AXIS2_PLACEMENT_3D ( 'NONE', #5073, #11297, #11190 ) ;
#17480=VERTEX_POINT ( 'NONE', #981 ) ;
#17483=ORIENTED_EDGE ( 'NONE', *, *, #6721, .F. ) ;
#17505=DIRECTION ( 'NONE',  ( 0.9396926207859112035, 0.3420201433256609969, -6.456589605409174593E-15 ) ) ;
#17513=ORIENTED_EDGE ( 'NONE', *, *, #17876, .F. ) ;
#17526=PRODUCT_CONTEXT ( 'NONE', #14162, 'mechanical' ) ;
#17535=DIRECTION ( 'NONE',  ( -6.982962677686266711E-15, 0.000000000000000000, -1.000000000000000000 ) ) ;
#17576=VERTEX_POINT ( 'NONE', #18693 ) ;
#17578=CARTESIAN_POINT ( 'NONE',  ( -1.396592535537253342E-14, 0.000000000000000000, 39.88498244535545467 ) ) ;
#17612=VECTOR ( 'NONE', #4667, 1000.000000000000000 ) ;
#17614=DIRECTION ( 'NONE',  ( 0.9396926207859057634, -0.3420201433256757073, -6.561838499445174030E-15 ) ) ;
#17618=ORIENTED_EDGE ( 'NONE', *, *, #11813, .T. ) ;
#17623=ORIENTED_EDGE ( 'NONE', *, *, #520, .T. ) ;
#17626=SHAPE_DEFINITION_REPRESENTATION ( #4755, #5472 ) ;
#17630=DIRECTION ( 'NONE',  ( -0.1736481776669273336, 0.9848077530122086864, 1.214091813839188063E-15 ) ) ;
#17638=CARTESIAN_POINT ( 'NONE',  ( -103.8888757476051836, -46.65403860089418941, 39.88498244535617943 ) ) ;
#17654=VECTOR ( 'NONE', #754, 1000.000000000000000 ) ;
#17657=DIRECTION ( 'NONE',  ( -6.982962677686266711E-15, 0.000000000000000000, -1.000000000000000000 ) ) ;
#17658=DIRECTION ( 'NONE',  ( 0.5000000000000039968, 0.8660254037844362651, -4.304393070272777803E-15 ) ) ;
#17667=ADVANCED_FACE ( 'NONE', ( #4207 ), #14756, .T. ) ;
#17679=CARTESIAN_POINT ( 'NONE',  ( 1.396592535537252080E-14, 0.000000000000000000, 49.99999999999998579 ) ) ;
#17681=DIRECTION ( 'NONE',  ( -1.000000000000000000, 0.000000000000000000, 6.969309079188926949E-15 ) ) ;
#17686=ORIENTED_EDGE ( 'NONE', *, *, #16188, .F. ) ;
#17696=AXIS2_PLACEMENT_3D ( 'NONE', #7523, #9367, #15611 ) ;
#17708=FACE_OUTER_BOUND ( 'NONE', #14849, .T. ) ;
#17720=ORIENTED_EDGE ( 'NONE', *, *, #6857, .T. ) ;
#17728=DIRECTION ( 'NONE',  ( -6.982962677686266711E-15, 0.000000000000000000, -1.000000000000000000 ) ) ;
#17731=DIRECTION ( 'NONE',  ( 6.982962677686266711E-15, 0.000000000000000000, 1.000000000000000000 ) ) ;
#17738=EDGE_CURVE ( 'NONE', #6114, #13453, #7088, .T. ) ;
#17743=ORIENTED_EDGE ( 'NONE', *, *, #18300, .T. ) ;
#17744=DIRECTION ( 'NONE',  ( -6.982962677686266711E-15, 0.000000000000000000, -1.000000000000000000 ) ) ;
#17752=EDGE_CURVE ( 'NONE', #15057, #10957, #8426, .T. ) ;
#17772=AXIS2_PLACEMENT_3D ( 'NONE', #3375, #11141, #19038 ) ;
#17783=CARTESIAN_POINT ( 'NONE',  ( -21.73104181959829617, -16.26654594725003733, 39.88498244535560389 ) ) ;
#17787=CARTESIAN_POINT ( 'NONE',  ( -63.98537287693041264, 94.20918150411493741, 14.88498244535589876 ) ) ;
#17789=ADVANCED_FACE ( 'NONE', ( #17002 ), #12384, .T. ) ;
#17795=ORIENTED_EDGE ( 'NONE', *, *, #12462, .T. ) ;
#17801=DIRECTION ( 'NONE',  ( 6.982962677686266711E-15, -0.000000000000000000, 1.000000000000000000 ) ) ;
#17819=AXIS2_PLACEMENT_3D ( 'NONE', #14919, #613, #6856 ) ;
#17820=ORIENTED_EDGE ( 'NONE', *, *, #19165, .F. ) ;
#17841=VERTEX_POINT ( 'NONE', #1553 ) ;
#17846=DIRECTION ( 'NONE',  ( -0.7660444431189770143, 0.6427876096865404731, 5.346191897317644012E-15 ) ) ;
#17876=EDGE_CURVE ( 'NONE', #15471, #7939, #4514, .T. ) ;
#17887=ADVANCED_FACE ( 'NONE', ( #15250 ), #1236, .T. ) ;
#17894=ORIENTED_EDGE ( 'NONE', *, *, #18504, .T. ) ;
#17898=CIRCLE ( 'NONE', #895, 106.4288957539801146 ) ;
#17901=ORIENTED_EDGE ( 'NONE', *, *, #11514, .F. ) ;
#17912=AXIS2_PLACEMENT_3D ( 'NONE', #9885, #13141, #17681 ) ;
#17913=ORIENTED_EDGE ( 'NONE', *, *, #6760, .F. ) ;
#17930=VERTEX_POINT ( 'NONE', #12691 ) ;
#17939=VERTEX_POINT ( 'NONE', #9532 ) ;
#17951=AXIS2_PLACEMENT_3D ( 'NONE', #239, #6492, #12713 ) ;
#17962=ORIENTED_EDGE ( 'NONE', *, *, #19303, .F. ) ;
#17965=ORIENTED_EDGE ( 'NONE', *, *, #19303, .T. ) ;
#17992=CARTESIAN_POINT ( 'NONE',  ( -113.3514208120935933, -17.29894464209964866, 39.88498244535624337 ) ) ;
#17994=AXIS2_PLACEMENT_3D ( 'NONE', #18003, #9923, #2159 ) ;
#17998=DIRECTION ( 'NONE',  ( 0.000000000000000000, 0.000000000000000000, 1.000000000000000000 ) ) ;
#18003=CARTESIAN_POINT ( 'NONE',  ( -63.98537287693041264, 94.20918150411493741, 14.88498244535589876 ) ) ;
#18017=EDGE_CURVE ( 'NONE', #4108, #7679, #2556, .T. ) ;
#18027=DIRECTION ( 'NONE',  ( -6.982962677686266711E-15, 0.000000000000000000, -1.000000000000000000 ) ) ;
#18031=DIRECTION ( 'NONE',  ( 0.000000000000000000, 0.000000000000000000, 1.000000000000000000 ) ) ;
#18032=DIRECTION ( 'NONE',  ( -6.982962677686266711E-15, 0.000000000000000000, -1.000000000000000000 ) ) ;
#18035=CARTESIAN_POINT ( 'NONE',  ( 14.85701326357409968, 22.71800723006099432, 14.88498244535534809 ) ) ;
#18052=AXIS2_PLACEMENT_3D ( 'NONE', #10530, #7369, #4406 ) ;
#18053=DIRECTION ( 'NONE',  ( 6.982962677686266711E-15, -0.000000000000000000, 1.000000000000000000 ) ) ;
#18083=AXIS2_PLACEMENT_3D ( 'NONE', #5865, #4423, #16805 ) ;
#18084=ORIENTED_EDGE ( 'NONE', *, *, #11209, .F. ) ;
#18092=CARTESIAN_POINT ( 'NONE',  ( -117.2142335457655520, -12.13581325405623268, 14.88498244535627002 ) ) ;
#18100=STYLED_ITEM ( 'NONE', ( #18292 ), #1084 ) ;
#18113=LINE ( 'NONE', #4087, #19239 ) ;
#18114=DIRECTION ( 'NONE',  ( 0.4999999999999916178, -0.8660254037844435926, -3.228294802704586902E-15 ) ) ;
#18123=CIRCLE ( 'NONE', #17819, 112.8770930172170210 ) ;
#18145=ADVANCED_FACE ( 'NONE', ( #5726 ), #10132, .T. ) ;
#18151=ORIENTED_EDGE ( 'NONE', *, *, #14769, .T. ) ;
#18158=DIRECTION ( 'NONE',  ( 0.9396926207859112035, 0.3420201433256609969, -6.456589605409174593E-15 ) ) ;
#18168=LINE ( 'NONE', #8852, #2504 ) ;
#18183=ORIENTED_EDGE ( 'NONE', *, *, #4401, .T. ) ;
#18203=ORIENTED_EDGE ( 'NONE', *, *, #10096, .T. ) ;
#18209=CARTESIAN_POINT ( 'NONE',  ( 81.66698895276879000, 79.37254397626031732, 14.88498244535488269 ) ) ;
#18211=VERTEX_POINT ( 'NONE', #15030 ) ;
#18219=ADVANCED_FACE ( 'NONE', ( #13689, #18509, #9088, #7656, #2860, #7452, #10416, #19933, #5938, #15329, #15224 ), #12359, .T. ) ;
#18236=DIRECTION ( 'NONE',  ( 6.982962677686266711E-15, -0.000000000000000000, 1.000000000000000000 ) ) ;
#18254=EDGE_LOOP ( 'NONE', ( #12484, #6008, #15186, #1760, #2024, #11891 ) ) ;
#18259=VECTOR ( 'NONE', #2880, 1000.000000000000000 ) ;
#18266=CARTESIAN_POINT ( 'NONE',  ( 1.396592535537252080E-14, 0.000000000000000000, 127.7817459305202448 ) ) ;
#18283=CARTESIAN_POINT ( 'NONE',  ( -109.5721339228235820, 31.03941509555038181, 39.88498244535622206 ) ) ;
#18292=PRESENTATION_STYLE_ASSIGNMENT (( #13982 ) ) ;
#18294=ORIENTED_EDGE ( 'NONE', *, *, #3991, .T. ) ;
#18300=EDGE_CURVE ( 'NONE', #14181, #10780, #2623, .T. ) ;
#18303=CYLINDRICAL_SURFACE ( 'NONE', #2214, 3.224098631618460331 ) ;
#18323=AXIS2_PLACEMENT_3D ( 'NONE', #15665, #3284, #15762 ) ;
#18330=ORIENTED_EDGE ( 'NONE', *, *, #19291, .F. ) ;
#18351=DIRECTION ( 'NONE',  ( 1.000000000000000000, 0.000000000000000000, -6.977185866873308817E-15 ) ) ;
#18365=AXIS2_PLACEMENT_3D ( 'NONE', #14661, #650, #18874 ) ;
#18391=AXIS2_PLACEMENT_3D ( 'NONE', #16791, #6985, #13202 ) ;
#18402=AXIS2_PLACEMENT_3D ( 'NONE', #10221, #5528, #13089 ) ;
#18411=DIRECTION ( 'NONE',  ( -1.000000000000000000, 0.000000000000000000, 6.982962677686266711E-15 ) ) ;
#18421=LINE ( 'NONE', #4397, #18739 ) ;
#18430=FACE_OUTER_BOUND ( 'NONE', #12101, .T. ) ;
#18452=CARTESIAN_POINT ( 'NONE',  ( -1.396592535537253342E-14, 0.000000000000000000, 39.88498244535545467 ) ) ;
#18460=ORIENTED_EDGE ( 'NONE', *, *, #6897, .F. ) ;
#18474=DIRECTION ( 'NONE',  ( 0.9396926207859104263, 0.3420201433256629397, -6.456589605409169071E-15 ) ) ;
#18482=LINE ( 'NONE', #15411, #19151 ) ;
#18484=AXIS2_PLACEMENT_3D ( 'NONE', #7243, #17801, #13462 ) ;
#18504=EDGE_CURVE ( 'NONE', #9562, #11829, #9049, .T. ) ;
#18506=DIRECTION ( 'NONE',  ( 1.000000000000000000, 0.000000000000000000, -6.976128451377902853E-15 ) ) ;
#18509=FACE_BOUND ( 'NONE', #10837, .T. ) ;
#18511=VERTEX_POINT ( 'NONE', #12114 ) ;
#18541=ORIENTED_EDGE ( 'NONE', *, *, #5358, .F. ) ;
#18543=ORIENTED_EDGE ( 'NONE', *, *, #9253, .T. ) ;
#18544=CARTESIAN_POINT ( 'NONE',  ( -2.647132857508373238, -114.6332882433608376, 39.88498244535547599 ) ) ;
#18564=ADVANCED_FACE ( 'NONE', ( #11303 ), #9469, .T. ) ;
#18569=FACE_OUTER_BOUND ( 'NONE', #8716, .T. ) ;
#18576=AXIS2_PLACEMENT_3D ( 'NONE', #13116, #17657, #11495 ) ;
#18580=AXIS2_PLACEMENT_3D ( 'NONE', #8085, #14339, #316 ) ;
#18583=CARTESIAN_POINT ( 'NONE',  ( 3.221721112346273674, 26.70531838198836283, 14.88498244535543158 ) ) ;
#18596=ORIENTED_EDGE ( 'NONE', *, *, #15257, .T. ) ;
#18602=DIRECTION ( 'NONE',  ( 6.982962677686266711E-15, 0.000000000000000000, 1.000000000000000000 ) ) ;
#18625=CIRCLE ( 'NONE', #8809, 3.224098631618459443 ) ;
#18628=CARTESIAN_POINT ( 'NONE',  ( -117.2142335457653672, -12.13581325405623268, 39.88498244535627180 ) ) ;
#18638=LINE ( 'NONE', #7778, #2700 ) ;
#18639=AXIS2_PLACEMENT_3D ( 'NONE', #8416, #18031, #13500 ) ;
#18650=EDGE_LOOP ( 'NONE', ( #3811, #18084, #9700, #17248 ) ) ;
#18651=EDGE_LOOP ( 'NONE', ( #6843, #1009, #6157, #2817 ) ) ;
#18668=CARTESIAN_POINT ( 'NONE',  ( -24.73834469112697576, -10.56256686379325593, 14.88498244535562520 ) ) ;
#18684=VERTEX_POINT ( 'NONE', #14676 ) ;
#18687=EDGE_CURVE ( 'NONE', #1807, #19254, #14678, .T. ) ;
#18691=DIRECTION ( 'NONE',  ( 6.982962677686266711E-15, -0.000000000000000000, 1.000000000000000000 ) ) ;
#18693=CARTESIAN_POINT ( 'NONE',  ( -23.19741967113651882, 4.658826548058537576, 39.88498244535561810 ) ) ;
#18695=ORIENTED_EDGE ( 'NONE', *, *, #2665, .T. ) ;
#18697=EDGE_LOOP ( 'NONE', ( #4783, #17290, #17720, #5450 ) ) ;
#18698=VERTEX_POINT ( 'NONE', #11786 ) ;
#18715=VECTOR ( 'NONE', #12790, 1000.000000000000000 ) ;
#18716=DIRECTION ( 'NONE',  ( 6.982962677686266711E-15, -0.000000000000000000, 1.000000000000000000 ) ) ;
#18722=CIRCLE ( 'NONE', #732, 106.4288957539801288 ) ;
#18723=ORIENTED_EDGE ( 'NONE', *, *, #18687, .T. ) ;
#18739=VECTOR ( 'NONE', #10623, 1000.000000000000000 ) ;
#18751=ORIENTED_EDGE ( 'NONE', *, *, #15121, .T. ) ;
#18754=EDGE_LOOP ( 'NONE', ( #14832, #9277, #4024, #5618 ) ) ;
#18785=DIRECTION ( 'NONE',  ( 6.982962677686266711E-15, 0.000000000000000000, 1.000000000000000000 ) ) ;
#18787=CYLINDRICAL_SURFACE ( 'NONE', #12806, 112.8770930172170210 ) ;
#18793=EDGE_CURVE ( 'NONE', #14390, #10728, #14015, .T. ) ;
#18809=DIRECTION ( 'NONE',  ( 6.982962677686266711E-15, 0.000000000000000000, 1.000000000000000000 ) ) ;
#18820=VECTOR ( 'NONE', #15097, 1000.000000000000000 ) ;
#18852=CIRCLE ( 'NONE', #19176, 3.224098631618461219 ) ;
#18874=DIRECTION ( 'NONE',  ( -0.1736481776669268895, 0.9848077530122086864, 1.076098267568195240E-15 ) ) ;
#18892=DIRECTION ( 'NONE',  ( -6.982962677686266711E-15, 0.000000000000000000, -1.000000000000000000 ) ) ;
#18903=ORIENTED_EDGE ( 'NONE', *, *, #10156, .T. ) ;
#18908=CYLINDRICAL_SURFACE ( 'NONE', #19381, 17.50000000000000355 ) ;
#18917=EDGE_CURVE ( 'NONE', #315, #2786, #3506, .T. ) ;
#18922=CARTESIAN_POINT ( 'NONE',  ( -3.143238168843667690, 31.03941509555038181, 14.88498244535547599 ) ) ;
#18934=ORIENTED_EDGE ( 'NONE', *, *, #7511, .T. ) ;
#18944=CIRCLE ( 'NONE', #14983, 3.224098631618458555 ) ;
#18950=CARTESIAN_POINT ( 'NONE',  ( 71.65703592476617700, -89.51573765728305432, 39.88498244535495019 ) ) ;
#18951=DIRECTION ( 'NONE',  ( 6.982962677686266711E-15, -0.000000000000000000, 1.000000000000000000 ) ) ;
#18966=LINE ( 'NONE', #16090, #15462 ) ;
#18975=LINE ( 'NONE', #14455, #13437 ) ;
#18985=EDGE_LOOP ( 'NONE', ( #16703, #15339, #15651, #17686, #17468 ) ) ;
#18991=EDGE_CURVE ( 'NONE', #10780, #12128, #2628, .T. ) ;
#18993=AXIS2_PLACEMENT_3D ( 'NONE', #6734, #19218, #11435 ) ;
#19007=VERTEX_POINT ( 'NONE', #11478 ) ;
#19009=PLANE ( 'NONE',  #1065 ) ;
#19015=FACE_OUTER_BOUND ( 'NONE', #8119, .T. ) ;
#19029=AXIS2_PLACEMENT_3D ( 'NONE', #19578, #5374, #11599 ) ;
#19031=EDGE_CURVE ( 'NONE', #12565, #11748, #10779, .T. ) ;
#19038=DIRECTION ( 'NONE',  ( 0.9396926207859063185, -0.3420201433256742640, -6.456589605409180904E-15 ) ) ;
#19043=CARTESIAN_POINT ( 'NONE',  ( -26.42151830275515323, 4.658826548058537576, 14.88498244535563586 ) ) ;
#19044=AXIS2_PLACEMENT_3D ( 'NONE', #5777, #2036, #692 ) ;
#19047=CARTESIAN_POINT ( 'NONE',  ( 27.90514497005375461, -110.4119590718113244, 14.88498244535525750 ) ) ;
#19052=DIRECTION ( 'NONE',  ( 1.000000000000000000, 0.000000000000000000, -6.969309079188926949E-15 ) ) ;
#19083=ORIENTED_EDGE ( 'NONE', *, *, #18504, .F. ) ;
#19103=EDGE_CURVE ( 'NONE', #17930, #10905, #16999, .T. ) ;
#19110=VERTEX_POINT ( 'NONE', #6885 ) ;
#19112=DIRECTION ( 'NONE',  ( -6.982962677686266711E-15, 0.000000000000000000, -1.000000000000000000 ) ) ;
#19114=EDGE_CURVE ( 'NONE', #19981, #6726, #640, .T. ) ;
#19122=DIRECTION ( 'NONE',  ( 6.982962677686266711E-15, -0.000000000000000000, 1.000000000000000000 ) ) ;
#19127=VERTEX_POINT ( 'NONE', #1024 ) ;
#19131=DIRECTION ( 'NONE',  ( 1.000000000000000000, 0.000000000000000000, 0.000000000000000000 ) ) ;
#19134=DIRECTION ( 'NONE',  ( -6.982962677686266711E-15, 0.000000000000000000, -1.000000000000000000 ) ) ;
#19136=DIRECTION ( 'NONE',  ( 6.982962677686266711E-15, -0.000000000000000000, 1.000000000000000000 ) ) ;
#19140=CIRCLE ( 'NONE', #12251, 3.224098631618458999 ) ;
#19151=VECTOR ( 'NONE', #5910, 1000.000000000000000 ) ;
#19152=ORIENTED_EDGE ( 'NONE', *, *, #15905, .F. ) ;
#19158=EDGE_LOOP ( 'NONE', ( #17371, #17423, #10568, #11377 ) ) ;
#19165=EDGE_CURVE ( 'NONE', #11748, #4614, #8176, .T. ) ;
#19176=AXIS2_PLACEMENT_3D ( 'NONE', #13867, #6215, #2832 ) ;
#19186=DIRECTION ( 'NONE',  ( -1.000000000000000000, 0.000000000000000000, 7.065055611250995019E-15 ) ) ;
#19197=CARTESIAN_POINT ( 'NONE',  ( -72.04228783541182679, 71.00759552807944885, 14.88498244535595560 ) ) ;
#19217=FACE_OUTER_BOUND ( 'NONE', #13676, .T. ) ;
#19218=DIRECTION ( 'NONE',  ( -6.982962677686266711E-15, 0.000000000000000000, -1.000000000000000000 ) ) ;
#19221=CARTESIAN_POINT ( 'NONE',  ( -63.98537287693023501, 94.20918150411493741, 39.88498244535590231 ) ) ;
#19224=EDGE_LOOP ( 'NONE', ( #8443, #17203, #5804, #9881, #6194, #2227 ) ) ;
#19236=DIRECTION ( 'NONE',  ( -6.982962677686266711E-15, 0.000000000000000000, -1.000000000000000000 ) ) ;
#19239=VECTOR ( 'NONE', #8892, 1000.000000000000000 ) ;
#19254=VERTEX_POINT ( 'NONE', #4823 ) ;
#19275=AXIS2_PLACEMENT_3D ( 'NONE', #10892, #17149, #3134 ) ;
#19284=ADVANCED_FACE ( 'NONE', ( #4716 ), #9619, .F. ) ;
#19286=DIRECTION ( 'NONE',  ( 1.000000000000000000, 0.000000000000000000, -6.976128451377902853E-15 ) ) ;
#19291=EDGE_CURVE ( 'NONE', #18211, #19007, #1647, .T. ) ;
#19303=EDGE_CURVE ( 'NONE', #1862, #12128, #612, .T. ) ;
#19310=DIRECTION ( 'NONE',  ( -0.7660444431189772363, 0.6427876096865402511, 5.380491337840974226E-15 ) ) ;
#19317=CARTESIAN_POINT ( 'NONE',  ( -97.59206265536059277, 66.04728469612305730, 39.88498244535613679 ) ) ;
#19319=DIRECTION ( 'NONE',  ( 6.982962677686266711E-15, 0.000000000000000000, 1.000000000000000000 ) ) ;
#19357=DIRECTION ( 'NONE',  ( -1.000000000000000000, 0.000000000000000000, 7.007922368489490773E-15 ) ) ;
#19360=DIRECTION ( 'NONE',  ( 6.982962677686266711E-15, -0.000000000000000000, 1.000000000000000000 ) ) ;
#19370=DIRECTION ( 'NONE',  ( -6.982962677686266711E-15, 0.000000000000000000, -1.000000000000000000 ) ) ;
#19376=ORIENTED_EDGE ( 'NONE', *, *, #15239, .T. ) ;
#19381=AXIS2_PLACEMENT_3D ( 'NONE', #17578, #16036, #6628 ) ;
#19385=DIRECTION ( 'NONE',  ( -6.982962677686266711E-15, 0.000000000000000000, -1.000000000000000000 ) ) ;
#19402=AXIS2_PLACEMENT_3D ( 'NONE', #10276, #9042, #18158 ) ;
#19416=ADVANCED_FACE ( 'NONE', ( #13374 ), #3684, .T. ) ;
#19422=DIRECTION ( 'NONE',  ( 6.982962677686266711E-15, -0.000000000000000000, 1.000000000000000000 ) ) ;
#19430=EDGE_LOOP ( 'NONE', ( #368, #9732, #18203, #13169 ) ) ;
#19435=CARTESIAN_POINT ( 'NONE',  ( 17.24542129382134803, 20.55229278271219329, 39.88498244535533388 ) ) ;
#19444=AXIS2_PLACEMENT_3D ( 'NONE', #7744, #18602, #6232 ) ;
#19459=ORIENTED_EDGE ( 'NONE', *, *, #9873, .F. ) ;
#19475=ORIENTED_EDGE ( 'NONE', *, *, #2050, .F. ) ;
#19476=CYLINDRICAL_SURFACE ( 'NONE', #3383, 106.4288957539801004 ) ;
#19480=DIRECTION ( 'NONE',  ( 0.4999999999999916178, -0.8660254037844435926, -3.228294802704586902E-15 ) ) ;
#19491=ORIENTED_EDGE ( 'NONE', *, *, #2782, .T. ) ;
#19499=DIRECTION ( 'NONE',  ( -6.982962677686266711E-15, 0.000000000000000000, -1.000000000000000000 ) ) ;
#19500=VERTEX_POINT ( 'NONE', #4564 ) ;
#19509=EDGE_CURVE ( 'NONE', #3202, #20085, #15714, .T. ) ;
#19520=EDGE_CURVE ( 'NONE', #11508, #10450, #1495, .T. ) ;
#19521=DIRECTION ( 'NONE',  ( 6.982962677686266711E-15, -0.000000000000000000, 1.000000000000000000 ) ) ;
#19525=CARTESIAN_POINT ( 'NONE',  ( 42.44352287704987248, 94.20918150411493741, 39.88498244535516335 ) ) ;
#19529=CARTESIAN_POINT ( 'NONE',  ( -14.69786621328411869, 22.52834316112731017, 14.88498244535555592 ) ) ;
#19532=DIRECTION ( 'NONE',  ( -6.982962677686266711E-15, 0.000000000000000000, -1.000000000000000000 ) ) ;
#19538=ORIENTED_EDGE ( 'NONE', *, *, #16197, .T. ) ;
#19551=EDGE_CURVE ( 'NONE', #15057, #8591, #59, .T. ) ;
#19558=VERTEX_POINT ( 'NONE', #19624 ) ;
#19578=CARTESIAN_POINT ( 'NONE',  ( 113.5802308907677372, 8.308367629983374414, 39.88498244535465886 ) ) ;
#19585=AXIS2_PLACEMENT_3D ( 'NONE', #11948, #10424, #3278 ) ;
#19624=CARTESIAN_POINT ( 'NONE',  ( 100.5989061668482520, 55.02415981988612970, 14.88498244535475123 ) ) ;
#19625=CARTESIAN_POINT ( 'NONE',  ( 3.221721112346273674, 26.70531838198836283, 14.88498244535543158 ) ) ;
#19629=ADVANCED_FACE ( 'NONE', ( #466, #1799 ), #259, .F. ) ;
#19653=DIRECTION ( 'NONE',  ( -0.7660444431189858960, -0.6427876096865299260, 5.346191897317643224E-15 ) ) ;
#19660=ORIENTED_EDGE ( 'NONE', *, *, #3964, .T. ) ;
#19670=DIRECTION ( 'NONE',  ( -6.982962677686266711E-15, 0.000000000000000000, -1.000000000000000000 ) ) ;
#19672=EDGE_LOOP ( 'NONE', ( #5996, #16553, #6242, #5474 ) ) ;
#19681=AXIS2_PLACEMENT_3D ( 'NONE', #11387, #2089, #2679 ) ;
#19684=ORIENTED_EDGE ( 'NONE', *, *, #14892, .T. ) ;
#19688=DIRECTION ( 'NONE',  ( 6.982962677686266711E-15, -0.000000000000000000, 1.000000000000000000 ) ) ;
#19701=EDGE_CURVE ( 'NONE', #8834, #6452, #568, .T. ) ;
#19703=VERTEX_POINT ( 'NONE', #8031 ) ;
#19716=EDGE_CURVE ( 'NONE', #17433, #18511, #12757, .T. ) ;
#19721=DIRECTION ( 'NONE',  ( 6.982962677686266711E-15, -0.000000000000000000, 1.000000000000000000 ) ) ;
#19725=FACE_OUTER_BOUND ( 'NONE', #9208, .T. ) ;
#19735=CIRCLE ( 'NONE', #9951, 3.224098631618460775 ) ;
#19756=CARTESIAN_POINT ( 'NONE',  ( -2.300765332208364988, -116.0870680293436408, 14.88498244535546711 ) ) ;
#19764=CIRCLE ( 'NONE', #19681, 3.224098631618458999 ) ;
#19787=ADVANCED_FACE ( 'NONE', ( #14773 ), #8437, .T. ) ;
#19789=AXIS2_PLACEMENT_3D ( 'NONE', #15238, #9099, #1225 ) ;
#19790=LINE ( 'NONE', #19987, #4058 ) ;
#19795=EDGE_CURVE ( 'NONE', #19254, #3116, #9174, .T. ) ;
#19801=CIRCLE ( 'NONE', #13584, 3.224098631618462552 ) ;
#19804=ORIENTED_EDGE ( 'NONE', *, *, #11291, .T. ) ;
#19806=DIRECTION ( 'NONE',  ( -6.982962677686266711E-15, 0.000000000000000000, -1.000000000000000000 ) ) ;
#19811=ORIENTED_EDGE ( 'NONE', *, *, #13333, .T. ) ;
#19820=AXIS2_PLACEMENT_3D ( 'NONE', #6264, #15872, #11359 ) ;
#19827=CARTESIAN_POINT ( 'NONE',  ( -100.8303968649779421, 8.087083979452582838, 14.88498244535615633 ) ) ;
#19834=CIRCLE ( 'NONE', #11020, 112.8770930172170353 ) ;
#19849=PLANE ( 'NONE',  #12162 ) ;
#19867=EDGE_CURVE ( 'NONE', #12798, #20089, #17024, .T. ) ;
#19918=FACE_OUTER_BOUND ( 'NONE', #15731, .T. ) ;
#19926=DIRECTION ( 'NONE',  ( 6.982962677686266711E-15, -0.000000000000000000, 1.000000000000000000 ) ) ;
#19933=FACE_BOUND ( 'NONE', #7019, .T. ) ;
#19934=DIRECTION ( 'NONE',  ( -6.982962677686266711E-15, 0.000000000000000000, -1.000000000000000000 ) ) ;
#19950=CARTESIAN_POINT ( 'NONE',  ( -97.95177330934008353, 59.60912842347561025, 39.88498244535613679 ) ) ;
#19951=CARTESIAN_POINT ( 'NONE',  ( -14.02132266220276691, 20.55229278271246329, 14.88498244535555060 ) ) ;
#19957=EDGE_LOOP ( 'NONE', ( #1411, #14639, #10829, #13194 ) ) ;
#19981=VERTEX_POINT ( 'NONE', #18668 ) ;
#19987=CARTESIAN_POINT ( 'NONE',  ( 106.5208805777952676, 53.25886146954521649, 14.88498244535470683 ) ) ;
#19993=EDGE_CURVE ( 'NONE', #13679, #6744, #16390, .T. ) ;
#20050=CIRCLE ( 'NONE', #6998, 112.8770930172170068 ) ;
#20085=VERTEX_POINT ( 'NONE', #138 ) ;
#20089=VERTEX_POINT ( 'NONE', #446 ) ;
#20092=ORIENTED_EDGE ( 'NONE', *, *, #14262, .F. ) ;
#20099=CYLINDRICAL_SURFACE ( 'NONE', #16330, 106.4288957539800862 ) ;
#20103=FACE_OUTER_BOUND ( 'NONE', #15389, .T. ) ;
#20133=DIRECTION ( 'NONE',  ( 1.000000000000000000, 0.000000000000000000, -6.994638739193269649E-15 ) ) ;
#20143=ORIENTED_EDGE ( 'NONE', *, *, #6760, .T. ) ;
#20151=ORIENTED_EDGE ( 'NONE', *, *, #8839, .F. ) ;
#20196=ORIENTED_EDGE ( 'NONE', *, *, #19551, .F. ) ;
#20205=VECTOR ( 'NONE', #5396, 1000.000000000000000 ) ;
#20207=CYLINDRICAL_SURFACE ( 'NONE', #19275, 127.4413876050234649 ) ;
#20218=ORIENTED_EDGE ( 'NONE', *, *, #15775, .F. ) ;
#20236=VECTOR ( 'NONE', #8131, 1000.000000000000000 ) ;
#20238=EDGE_CURVE ( 'NONE', #17480, #9831, #11752, .T. ) ;
ENDSEC;
END-ISO-10303-21;
